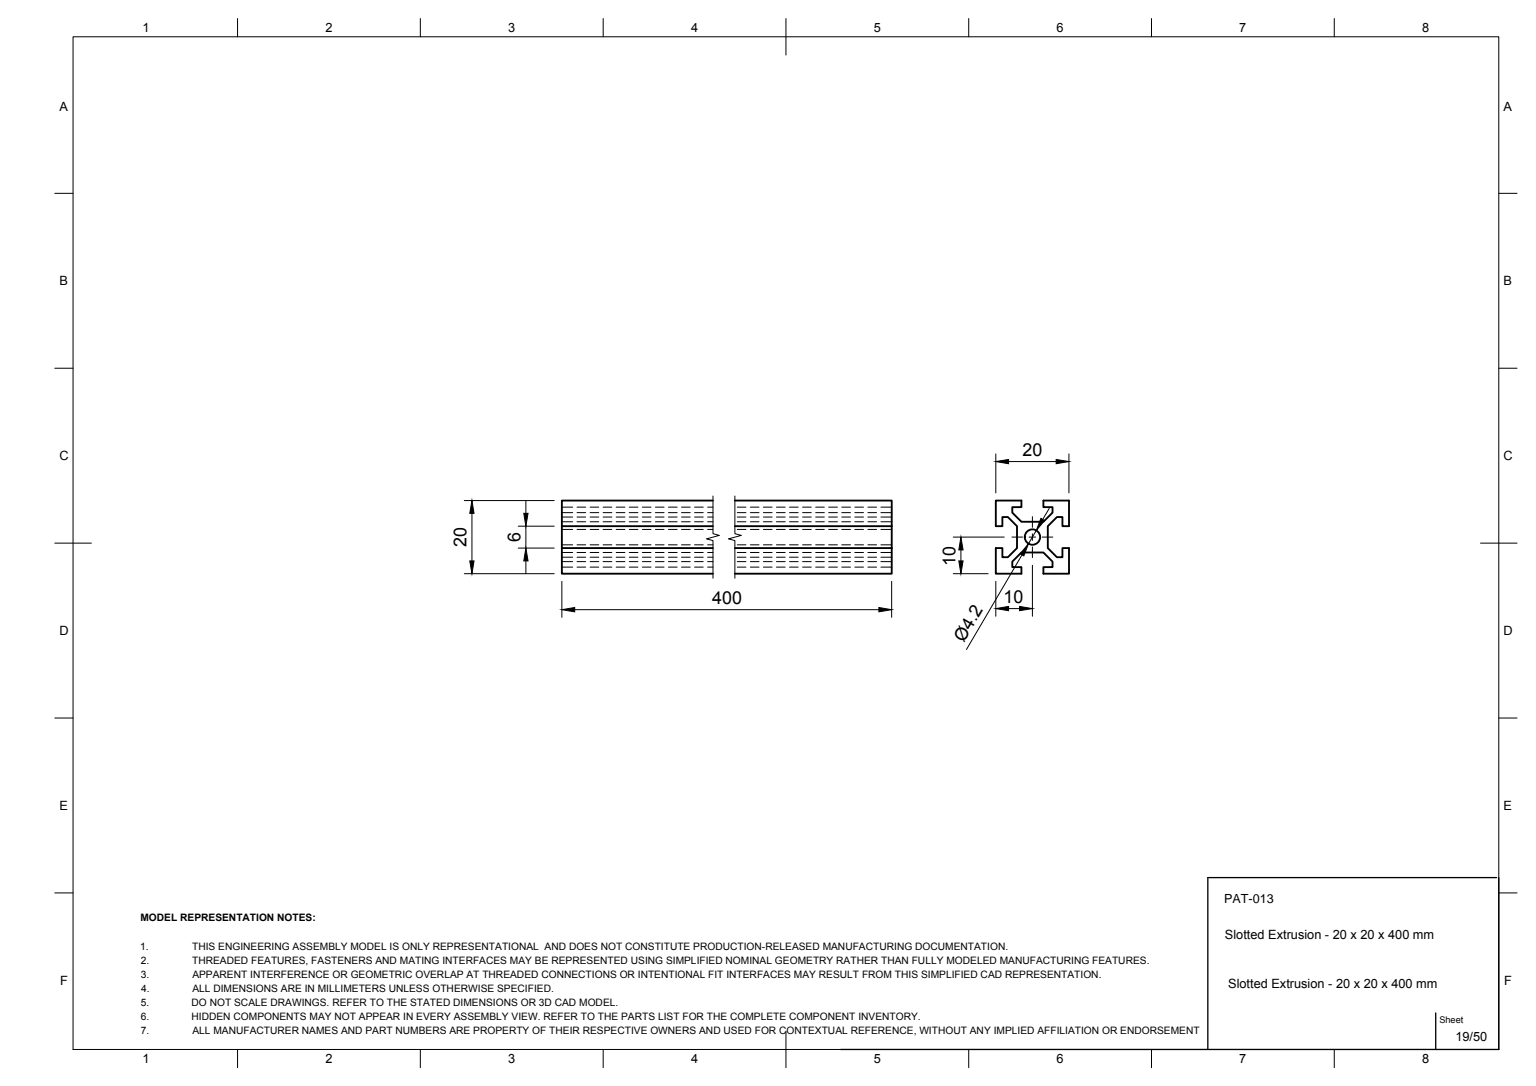
ISO-10303-21;
HEADER;
/* Generated by software containing ST-Developer
 * from STEP Tools, Inc. (www.steptools.com) 
 */

FILE_DESCRIPTION(
/* description */ ('Belt-driven linear axis on 2020 extrusion'),
/* implementation_level */ '2;1');

FILE_NAME(
/* name */ 'Slotted Extrusion - 20 x 20 x 400 mm.step',
/* time_stamp */ '2026-10-28T03:26:09-07:00',
/* author */ (''),
/* organization */ (''),
/* preprocessor_version */ 'ST-DEVELOPER v20.2',
/* originating_system */ 'Autodesk Translation Framework v15.17.0.0',
/* authorisation */ '');

FILE_SCHEMA (('AUTOMOTIVE_DESIGN { 1 0 10303 214 3 1 1 }'));
ENDSEC;

DATA;
#10=MECHANICAL_DESIGN_GEOMETRIC_PRESENTATION_REPRESENTATION('',(#639),#20096);
#537=SHAPE_REPRESENTATION_RELATIONSHIP('SRR','None',#20334,#583);
#583=ADVANCED_BREP_SHAPE_REPRESENTATION('',(#695),#20065);
#639=STYLED_ITEM('',(#20636),#695);
#695=MANIFOLD_SOLID_BREP('Body1',#10952);
#813=FACE_BOUND('',#2278,.T.);
#814=FACE_BOUND('',#2280,.T.);
#1022=PLANE('',#12051);
#1023=PLANE('',#12052);
#1024=PLANE('',#12053);
#1025=PLANE('',#12054);
#1026=PLANE('',#12055);
#1027=PLANE('',#12056);
#1028=PLANE('',#12057);
#1029=PLANE('',#12058);
#1030=PLANE('',#12059);
#1031=PLANE('',#12060);
#1032=PLANE('',#12061);
#1033=PLANE('',#12062);
#1034=PLANE('',#12063);
#1035=PLANE('',#12064);
#1036=PLANE('',#12065);
#1037=PLANE('',#12066);
#1038=PLANE('',#12067);
#1039=PLANE('',#12068);
#1040=PLANE('',#12069);
#1041=PLANE('',#12070);
#1042=PLANE('',#12071);
#1043=PLANE('',#12072);
#1044=PLANE('',#12073);
#1045=PLANE('',#12074);
#1046=PLANE('',#12075);
#1047=PLANE('',#12076);
#1048=PLANE('',#12077);
#1049=PLANE('',#12078);
#1050=PLANE('',#12079);
#1051=PLANE('',#12080);
#1052=PLANE('',#12081);
#1053=PLANE('',#12082);
#1054=PLANE('',#12083);
#1055=PLANE('',#12084);
#1056=PLANE('',#12085);
#1057=PLANE('',#12086);
#1058=PLANE('',#12090);
#1059=PLANE('',#12091);
#1060=PLANE('',#12092);
#1061=PLANE('',#12093);
#1062=PLANE('',#12094);
#1063=PLANE('',#12095);
#1064=PLANE('',#12096);
#1065=PLANE('',#12097);
#1066=PLANE('',#12098);
#1067=PLANE('',#12099);
#1515=FACE_OUTER_BOUND('',#2232,.T.);
#1516=FACE_OUTER_BOUND('',#2233,.T.);
#1517=FACE_OUTER_BOUND('',#2234,.T.);
#1518=FACE_OUTER_BOUND('',#2235,.T.);
#1519=FACE_OUTER_BOUND('',#2236,.T.);
#1520=FACE_OUTER_BOUND('',#2237,.T.);
#1521=FACE_OUTER_BOUND('',#2238,.T.);
#1522=FACE_OUTER_BOUND('',#2239,.T.);
#1523=FACE_OUTER_BOUND('',#2240,.T.);
#1524=FACE_OUTER_BOUND('',#2241,.T.);
#1525=FACE_OUTER_BOUND('',#2242,.T.);
#1526=FACE_OUTER_BOUND('',#2243,.T.);
#1527=FACE_OUTER_BOUND('',#2244,.T.);
#1528=FACE_OUTER_BOUND('',#2245,.T.);
#1529=FACE_OUTER_BOUND('',#2246,.T.);
#1530=FACE_OUTER_BOUND('',#2247,.T.);
#1531=FACE_OUTER_BOUND('',#2248,.T.);
#1532=FACE_OUTER_BOUND('',#2249,.T.);
#1533=FACE_OUTER_BOUND('',#2250,.T.);
#1534=FACE_OUTER_BOUND('',#2251,.T.);
#1535=FACE_OUTER_BOUND('',#2252,.T.);
#1536=FACE_OUTER_BOUND('',#2253,.T.);
#1537=FACE_OUTER_BOUND('',#2254,.T.);
#1538=FACE_OUTER_BOUND('',#2255,.T.);
#1539=FACE_OUTER_BOUND('',#2256,.T.);
#1540=FACE_OUTER_BOUND('',#2257,.T.);
#1541=FACE_OUTER_BOUND('',#2258,.T.);
#1542=FACE_OUTER_BOUND('',#2259,.T.);
#1543=FACE_OUTER_BOUND('',#2260,.T.);
#1544=FACE_OUTER_BOUND('',#2261,.T.);
#1545=FACE_OUTER_BOUND('',#2262,.T.);
#1546=FACE_OUTER_BOUND('',#2263,.T.);
#1547=FACE_OUTER_BOUND('',#2264,.T.);
#1548=FACE_OUTER_BOUND('',#2265,.T.);
#1549=FACE_OUTER_BOUND('',#2266,.T.);
#1550=FACE_OUTER_BOUND('',#2267,.T.);
#1551=FACE_OUTER_BOUND('',#2268,.T.);
#1552=FACE_OUTER_BOUND('',#2269,.T.);
#1553=FACE_OUTER_BOUND('',#2270,.T.);
#1554=FACE_OUTER_BOUND('',#2271,.T.);
#1555=FACE_OUTER_BOUND('',#2272,.T.);
#1556=FACE_OUTER_BOUND('',#2273,.T.);
#1557=FACE_OUTER_BOUND('',#2274,.T.);
#1558=FACE_OUTER_BOUND('',#2275,.T.);
#1559=FACE_OUTER_BOUND('',#2276,.T.);
#1560=FACE_OUTER_BOUND('',#2277,.T.);
#1561=FACE_OUTER_BOUND('',#2279,.T.);
#2232=EDGE_LOOP('',(#8437,#8438,#8439,#8440));
#2233=EDGE_LOOP('',(#8441,#8442,#8443,#8444));
#2234=EDGE_LOOP('',(#8445,#8446,#8447,#8448));
#2235=EDGE_LOOP('',(#8449,#8450,#8451,#8452));
#2236=EDGE_LOOP('',(#8453,#8454,#8455,#8456));
#2237=EDGE_LOOP('',(#8457,#8458,#8459,#8460));
#2238=EDGE_LOOP('',(#8461,#8462,#8463,#8464));
#2239=EDGE_LOOP('',(#8465,#8466,#8467,#8468));
#2240=EDGE_LOOP('',(#8469,#8470,#8471,#8472));
#2241=EDGE_LOOP('',(#8473,#8474,#8475,#8476));
#2242=EDGE_LOOP('',(#8477,#8478,#8479,#8480));
#2243=EDGE_LOOP('',(#8481,#8482,#8483,#8484));
#2244=EDGE_LOOP('',(#8485,#8486,#8487,#8488));
#2245=EDGE_LOOP('',(#8489,#8490,#8491,#8492));
#2246=EDGE_LOOP('',(#8493,#8494,#8495,#8496));
#2247=EDGE_LOOP('',(#8497,#8498,#8499,#8500));
#2248=EDGE_LOOP('',(#8501,#8502,#8503,#8504));
#2249=EDGE_LOOP('',(#8505,#8506,#8507,#8508));
#2250=EDGE_LOOP('',(#8509,#8510,#8511,#8512));
#2251=EDGE_LOOP('',(#8513,#8514,#8515,#8516));
#2252=EDGE_LOOP('',(#8517,#8518,#8519,#8520));
#2253=EDGE_LOOP('',(#8521,#8522,#8523,#8524));
#2254=EDGE_LOOP('',(#8525,#8526,#8527,#8528));
#2255=EDGE_LOOP('',(#8529,#8530,#8531,#8532));
#2256=EDGE_LOOP('',(#8533,#8534,#8535,#8536));
#2257=EDGE_LOOP('',(#8537,#8538,#8539,#8540));
#2258=EDGE_LOOP('',(#8541,#8542,#8543,#8544));
#2259=EDGE_LOOP('',(#8545,#8546,#8547,#8548));
#2260=EDGE_LOOP('',(#8549,#8550,#8551,#8552));
#2261=EDGE_LOOP('',(#8553,#8554,#8555,#8556));
#2262=EDGE_LOOP('',(#8557,#8558,#8559,#8560));
#2263=EDGE_LOOP('',(#8561,#8562,#8563,#8564));
#2264=EDGE_LOOP('',(#8565,#8566,#8567,#8568));
#2265=EDGE_LOOP('',(#8569,#8570,#8571,#8572));
#2266=EDGE_LOOP('',(#8573,#8574,#8575,#8576));
#2267=EDGE_LOOP('',(#8577,#8578,#8579,#8580));
#2268=EDGE_LOOP('',(#8581,#8582,#8583,#8584));
#2269=EDGE_LOOP('',(#8585,#8586,#8587,#8588));
#2270=EDGE_LOOP('',(#8589,#8590,#8591,#8592));
#2271=EDGE_LOOP('',(#8593,#8594,#8595,#8596));
#2272=EDGE_LOOP('',(#8597,#8598,#8599,#8600));
#2273=EDGE_LOOP('',(#8601,#8602,#8603,#8604));
#2274=EDGE_LOOP('',(#8605,#8606,#8607,#8608));
#2275=EDGE_LOOP('',(#8609,#8610,#8611,#8612));
#2276=EDGE_LOOP('',(#8613,#8614,#8615,#8616));
#2277=EDGE_LOOP('',(#8617,#8618,#8619,#8620,#8621,#8622,#8623,#8624,#8625,
#8626,#8627,#8628,#8629,#8630,#8631,#8632,#8633,#8634,#8635,#8636,#8637,
#8638,#8639,#8640,#8641,#8642,#8643,#8644,#8645,#8646,#8647,#8648,#8649,
#8650,#8651,#8652,#8653,#8654,#8655,#8656,#8657,#8658,#8659,#8660));
#2278=EDGE_LOOP('',(#8661));
#2279=EDGE_LOOP('',(#8662,#8663,#8664,#8665,#8666,#8667,#8668,#8669,#8670,
#8671,#8672,#8673,#8674,#8675,#8676,#8677,#8678,#8679,#8680,#8681,#8682,
#8683,#8684,#8685,#8686,#8687,#8688,#8689,#8690,#8691,#8692,#8693,#8694,
#8695,#8696,#8697,#8698,#8699,#8700,#8701,#8702,#8703,#8704,#8705));
#2280=EDGE_LOOP('',(#8706));
#2971=LINE('',#17862,#3828);
#2972=LINE('',#17864,#3829);
#2973=LINE('',#17866,#3830);
#2974=LINE('',#17867,#3831);
#2975=LINE('',#17870,#3832);
#2976=LINE('',#17872,#3833);
#2977=LINE('',#17873,#3834);
#2978=LINE('',#17876,#3835);
#2979=LINE('',#17878,#3836);
#2980=LINE('',#17879,#3837);
#2981=LINE('',#17882,#3838);
#2982=LINE('',#17884,#3839);
#2983=LINE('',#17885,#3840);
#2984=LINE('',#17888,#3841);
#2985=LINE('',#17890,#3842);
#2986=LINE('',#17891,#3843);
#2987=LINE('',#17894,#3844);
#2988=LINE('',#17896,#3845);
#2989=LINE('',#17897,#3846);
#2990=LINE('',#17900,#3847);
#2991=LINE('',#17902,#3848);
#2992=LINE('',#17903,#3849);
#2993=LINE('',#17906,#3850);
#2994=LINE('',#17908,#3851);
#2995=LINE('',#17909,#3852);
#2996=LINE('',#17912,#3853);
#2997=LINE('',#17914,#3854);
#2998=LINE('',#17915,#3855);
#2999=LINE('',#17919,#3856);
#3000=LINE('',#17921,#3857);
#3001=LINE('',#17923,#3858);
#3002=LINE('',#17924,#3859);
#3003=LINE('',#17927,#3860);
#3004=LINE('',#17929,#3861);
#3005=LINE('',#17930,#3862);
#3006=LINE('',#17933,#3863);
#3007=LINE('',#17935,#3864);
#3008=LINE('',#17936,#3865);
#3009=LINE('',#17939,#3866);
#3010=LINE('',#17941,#3867);
#3011=LINE('',#17942,#3868);
#3012=LINE('',#17945,#3869);
#3013=LINE('',#17947,#3870);
#3014=LINE('',#17948,#3871);
#3015=LINE('',#17951,#3872);
#3016=LINE('',#17953,#3873);
#3017=LINE('',#17954,#3874);
#3018=LINE('',#17957,#3875);
#3019=LINE('',#17959,#3876);
#3020=LINE('',#17960,#3877);
#3021=LINE('',#17963,#3878);
#3022=LINE('',#17965,#3879);
#3023=LINE('',#17966,#3880);
#3024=LINE('',#17969,#3881);
#3025=LINE('',#17971,#3882);
#3026=LINE('',#17972,#3883);
#3027=LINE('',#17976,#3884);
#3028=LINE('',#17978,#3885);
#3029=LINE('',#17980,#3886);
#3030=LINE('',#17981,#3887);
#3031=LINE('',#17984,#3888);
#3032=LINE('',#17986,#3889);
#3033=LINE('',#17987,#3890);
#3034=LINE('',#17990,#3891);
#3035=LINE('',#17992,#3892);
#3036=LINE('',#17993,#3893);
#3037=LINE('',#17996,#3894);
#3038=LINE('',#17998,#3895);
#3039=LINE('',#17999,#3896);
#3040=LINE('',#18002,#3897);
#3041=LINE('',#18004,#3898);
#3042=LINE('',#18005,#3899);
#3043=LINE('',#18008,#3900);
#3044=LINE('',#18010,#3901);
#3045=LINE('',#18011,#3902);
#3046=LINE('',#18014,#3903);
#3047=LINE('',#18016,#3904);
#3048=LINE('',#18017,#3905);
#3049=LINE('',#18020,#3906);
#3050=LINE('',#18022,#3907);
#3051=LINE('',#18023,#3908);
#3052=LINE('',#18026,#3909);
#3053=LINE('',#18028,#3910);
#3054=LINE('',#18029,#3911);
#3055=LINE('',#18033,#3912);
#3056=LINE('',#18035,#3913);
#3057=LINE('',#18037,#3914);
#3058=LINE('',#18038,#3915);
#3059=LINE('',#18041,#3916);
#3060=LINE('',#18043,#3917);
#3061=LINE('',#18044,#3918);
#3062=LINE('',#18047,#3919);
#3063=LINE('',#18049,#3920);
#3064=LINE('',#18050,#3921);
#3065=LINE('',#18053,#3922);
#3066=LINE('',#18055,#3923);
#3067=LINE('',#18056,#3924);
#3068=LINE('',#18059,#3925);
#3069=LINE('',#18061,#3926);
#3070=LINE('',#18062,#3927);
#3071=LINE('',#18065,#3928);
#3072=LINE('',#18067,#3929);
#3073=LINE('',#18068,#3930);
#3074=LINE('',#18071,#3931);
#3075=LINE('',#18073,#3932);
#3076=LINE('',#18074,#3933);
#3077=LINE('',#18077,#3934);
#3078=LINE('',#18079,#3935);
#3079=LINE('',#18080,#3936);
#3080=LINE('',#18083,#3937);
#3081=LINE('',#18085,#3938);
#3082=LINE('',#18086,#3939);
#3083=LINE('',#18091,#3940);
#3084=LINE('',#18095,#3941);
#3085=LINE('',#18097,#3942);
#3086=LINE('',#18098,#3943);
#3087=LINE('',#18101,#3944);
#3088=LINE('',#18103,#3945);
#3089=LINE('',#18104,#3946);
#3090=LINE('',#18106,#3947);
#3091=LINE('',#18107,#3948);
#3092=LINE('',#18110,#3949);
#3093=LINE('',#18112,#3950);
#3094=LINE('',#18113,#3951);
#3095=LINE('',#18115,#3952);
#3096=LINE('',#18116,#3953);
#3097=LINE('',#18119,#3954);
#3098=LINE('',#18121,#3955);
#3099=LINE('',#18122,#3956);
#3100=LINE('',#18124,#3957);
#3101=LINE('',#18125,#3958);
#3102=LINE('',#18127,#3959);
#3103=LINE('',#18128,#3960);
#3828=VECTOR('',#14215,1.);
#3829=VECTOR('',#14216,1.);
#3830=VECTOR('',#14217,1.);
#3831=VECTOR('',#14218,1.);
#3832=VECTOR('',#14221,1.);
#3833=VECTOR('',#14222,1.);
#3834=VECTOR('',#14223,1.);
#3835=VECTOR('',#14226,1.);
#3836=VECTOR('',#14227,1.);
#3837=VECTOR('',#14228,1.);
#3838=VECTOR('',#14231,1.);
#3839=VECTOR('',#14232,1.);
#3840=VECTOR('',#14233,1.);
#3841=VECTOR('',#14236,1.);
#3842=VECTOR('',#14237,1.);
#3843=VECTOR('',#14238,1.);
#3844=VECTOR('',#14241,1.);
#3845=VECTOR('',#14242,1.);
#3846=VECTOR('',#14243,1.);
#3847=VECTOR('',#14246,1.);
#3848=VECTOR('',#14247,1.);
#3849=VECTOR('',#14248,1.);
#3850=VECTOR('',#14251,1.);
#3851=VECTOR('',#14252,1.);
#3852=VECTOR('',#14253,1.);
#3853=VECTOR('',#14256,1.);
#3854=VECTOR('',#14257,1.);
#3855=VECTOR('',#14258,1.);
#3856=VECTOR('',#14261,1.);
#3857=VECTOR('',#14262,1.);
#3858=VECTOR('',#14263,1.);
#3859=VECTOR('',#14264,1.);
#3860=VECTOR('',#14267,1.);
#3861=VECTOR('',#14268,1.);
#3862=VECTOR('',#14269,1.);
#3863=VECTOR('',#14272,1.);
#3864=VECTOR('',#14273,1.);
#3865=VECTOR('',#14274,1.);
#3866=VECTOR('',#14277,1.);
#3867=VECTOR('',#14278,1.);
#3868=VECTOR('',#14279,1.);
#3869=VECTOR('',#14282,1.);
#3870=VECTOR('',#14283,1.);
#3871=VECTOR('',#14284,1.);
#3872=VECTOR('',#14287,1.);
#3873=VECTOR('',#14288,1.);
#3874=VECTOR('',#14289,1.);
#3875=VECTOR('',#14292,1.);
#3876=VECTOR('',#14293,1.);
#3877=VECTOR('',#14294,1.);
#3878=VECTOR('',#14297,1.);
#3879=VECTOR('',#14298,1.);
#3880=VECTOR('',#14299,1.);
#3881=VECTOR('',#14302,1.);
#3882=VECTOR('',#14303,1.);
#3883=VECTOR('',#14304,1.);
#3884=VECTOR('',#14307,1.);
#3885=VECTOR('',#14308,1.);
#3886=VECTOR('',#14309,1.);
#3887=VECTOR('',#14310,1.);
#3888=VECTOR('',#14313,1.);
#3889=VECTOR('',#14314,1.);
#3890=VECTOR('',#14315,1.);
#3891=VECTOR('',#14318,1.);
#3892=VECTOR('',#14319,1.);
#3893=VECTOR('',#14320,1.);
#3894=VECTOR('',#14323,1.);
#3895=VECTOR('',#14324,1.);
#3896=VECTOR('',#14325,1.);
#3897=VECTOR('',#14328,1.);
#3898=VECTOR('',#14329,1.);
#3899=VECTOR('',#14330,1.);
#3900=VECTOR('',#14333,1.);
#3901=VECTOR('',#14334,1.);
#3902=VECTOR('',#14335,1.);
#3903=VECTOR('',#14338,1.);
#3904=VECTOR('',#14339,1.);
#3905=VECTOR('',#14340,1.);
#3906=VECTOR('',#14343,1.);
#3907=VECTOR('',#14344,1.);
#3908=VECTOR('',#14345,1.);
#3909=VECTOR('',#14348,1.);
#3910=VECTOR('',#14349,1.);
#3911=VECTOR('',#14350,1.);
#3912=VECTOR('',#14353,1.);
#3913=VECTOR('',#14354,1.);
#3914=VECTOR('',#14355,1.);
#3915=VECTOR('',#14356,1.);
#3916=VECTOR('',#14359,1.);
#3917=VECTOR('',#14360,1.);
#3918=VECTOR('',#14361,1.);
#3919=VECTOR('',#14364,1.);
#3920=VECTOR('',#14365,1.);
#3921=VECTOR('',#14366,1.);
#3922=VECTOR('',#14369,1.);
#3923=VECTOR('',#14370,1.);
#3924=VECTOR('',#14371,1.);
#3925=VECTOR('',#14374,1.);
#3926=VECTOR('',#14375,1.);
#3927=VECTOR('',#14376,1.);
#3928=VECTOR('',#14379,1.);
#3929=VECTOR('',#14380,1.);
#3930=VECTOR('',#14381,1.);
#3931=VECTOR('',#14384,1.);
#3932=VECTOR('',#14385,1.);
#3933=VECTOR('',#14386,1.);
#3934=VECTOR('',#14389,1.);
#3935=VECTOR('',#14390,1.);
#3936=VECTOR('',#14391,1.);
#3937=VECTOR('',#14394,1.);
#3938=VECTOR('',#14395,1.);
#3939=VECTOR('',#14396,1.);
#3940=VECTOR('',#14401,0.21);
#3941=VECTOR('',#14406,1.);
#3942=VECTOR('',#14407,1.);
#3943=VECTOR('',#14408,1.);
#3944=VECTOR('',#14411,1.);
#3945=VECTOR('',#14412,1.);
#3946=VECTOR('',#14413,1.);
#3947=VECTOR('',#14416,1.);
#3948=VECTOR('',#14417,1.);
#3949=VECTOR('',#14420,1.);
#3950=VECTOR('',#14421,1.);
#3951=VECTOR('',#14422,1.);
#3952=VECTOR('',#14425,1.);
#3953=VECTOR('',#14426,1.);
#3954=VECTOR('',#14429,1.);
#3955=VECTOR('',#14430,1.);
#3956=VECTOR('',#14431,1.);
#3957=VECTOR('',#14434,1.);
#3958=VECTOR('',#14435,1.);
#3959=VECTOR('',#14438,1.);
#3960=VECTOR('',#14439,1.);
#4647=CIRCLE('',#12088,0.21);
#4648=CIRCLE('',#12089,0.21);
#5296=VERTEX_POINT('',#17860);
#5297=VERTEX_POINT('',#17861);
#5298=VERTEX_POINT('',#17863);
#5299=VERTEX_POINT('',#17865);
#5300=VERTEX_POINT('',#17869);
#5301=VERTEX_POINT('',#17871);
#5302=VERTEX_POINT('',#17875);
#5303=VERTEX_POINT('',#17877);
#5304=VERTEX_POINT('',#17881);
#5305=VERTEX_POINT('',#17883);
#5306=VERTEX_POINT('',#17887);
#5307=VERTEX_POINT('',#17889);
#5308=VERTEX_POINT('',#17893);
#5309=VERTEX_POINT('',#17895);
#5310=VERTEX_POINT('',#17899);
#5311=VERTEX_POINT('',#17901);
#5312=VERTEX_POINT('',#17905);
#5313=VERTEX_POINT('',#17907);
#5314=VERTEX_POINT('',#17911);
#5315=VERTEX_POINT('',#17913);
#5316=VERTEX_POINT('',#17917);
#5317=VERTEX_POINT('',#17918);
#5318=VERTEX_POINT('',#17920);
#5319=VERTEX_POINT('',#17922);
#5320=VERTEX_POINT('',#17926);
#5321=VERTEX_POINT('',#17928);
#5322=VERTEX_POINT('',#17932);
#5323=VERTEX_POINT('',#17934);
#5324=VERTEX_POINT('',#17938);
#5325=VERTEX_POINT('',#17940);
#5326=VERTEX_POINT('',#17944);
#5327=VERTEX_POINT('',#17946);
#5328=VERTEX_POINT('',#17950);
#5329=VERTEX_POINT('',#17952);
#5330=VERTEX_POINT('',#17956);
#5331=VERTEX_POINT('',#17958);
#5332=VERTEX_POINT('',#17962);
#5333=VERTEX_POINT('',#17964);
#5334=VERTEX_POINT('',#17968);
#5335=VERTEX_POINT('',#17970);
#5336=VERTEX_POINT('',#17974);
#5337=VERTEX_POINT('',#17975);
#5338=VERTEX_POINT('',#17977);
#5339=VERTEX_POINT('',#17979);
#5340=VERTEX_POINT('',#17983);
#5341=VERTEX_POINT('',#17985);
#5342=VERTEX_POINT('',#17989);
#5343=VERTEX_POINT('',#17991);
#5344=VERTEX_POINT('',#17995);
#5345=VERTEX_POINT('',#17997);
#5346=VERTEX_POINT('',#18001);
#5347=VERTEX_POINT('',#18003);
#5348=VERTEX_POINT('',#18007);
#5349=VERTEX_POINT('',#18009);
#5350=VERTEX_POINT('',#18013);
#5351=VERTEX_POINT('',#18015);
#5352=VERTEX_POINT('',#18019);
#5353=VERTEX_POINT('',#18021);
#5354=VERTEX_POINT('',#18025);
#5355=VERTEX_POINT('',#18027);
#5356=VERTEX_POINT('',#18031);
#5357=VERTEX_POINT('',#18032);
#5358=VERTEX_POINT('',#18034);
#5359=VERTEX_POINT('',#18036);
#5360=VERTEX_POINT('',#18040);
#5361=VERTEX_POINT('',#18042);
#5362=VERTEX_POINT('',#18046);
#5363=VERTEX_POINT('',#18048);
#5364=VERTEX_POINT('',#18052);
#5365=VERTEX_POINT('',#18054);
#5366=VERTEX_POINT('',#18058);
#5367=VERTEX_POINT('',#18060);
#5368=VERTEX_POINT('',#18064);
#5369=VERTEX_POINT('',#18066);
#5370=VERTEX_POINT('',#18070);
#5371=VERTEX_POINT('',#18072);
#5372=VERTEX_POINT('',#18076);
#5373=VERTEX_POINT('',#18078);
#5374=VERTEX_POINT('',#18082);
#5375=VERTEX_POINT('',#18084);
#5376=VERTEX_POINT('',#18088);
#5377=VERTEX_POINT('',#18090);
#5378=VERTEX_POINT('',#18094);
#5379=VERTEX_POINT('',#18096);
#5380=VERTEX_POINT('',#18100);
#5381=VERTEX_POINT('',#18102);
#5382=VERTEX_POINT('',#18109);
#5383=VERTEX_POINT('',#18111);
#5384=VERTEX_POINT('',#18118);
#5385=VERTEX_POINT('',#18120);
#6433=EDGE_CURVE('',#5296,#5297,#2971,.T.);
#6434=EDGE_CURVE('',#5296,#5298,#2972,.T.);
#6435=EDGE_CURVE('',#5299,#5298,#2973,.T.);
#6436=EDGE_CURVE('',#5297,#5299,#2974,.T.);
#6437=EDGE_CURVE('',#5300,#5296,#2975,.T.);
#6438=EDGE_CURVE('',#5300,#5301,#2976,.T.);
#6439=EDGE_CURVE('',#5298,#5301,#2977,.T.);
#6440=EDGE_CURVE('',#5302,#5300,#2978,.T.);
#6441=EDGE_CURVE('',#5302,#5303,#2979,.T.);
#6442=EDGE_CURVE('',#5301,#5303,#2980,.T.);
#6443=EDGE_CURVE('',#5304,#5302,#2981,.T.);
#6444=EDGE_CURVE('',#5304,#5305,#2982,.T.);
#6445=EDGE_CURVE('',#5303,#5305,#2983,.T.);
#6446=EDGE_CURVE('',#5306,#5304,#2984,.T.);
#6447=EDGE_CURVE('',#5306,#5307,#2985,.T.);
#6448=EDGE_CURVE('',#5305,#5307,#2986,.T.);
#6449=EDGE_CURVE('',#5308,#5306,#2987,.T.);
#6450=EDGE_CURVE('',#5308,#5309,#2988,.T.);
#6451=EDGE_CURVE('',#5307,#5309,#2989,.T.);
#6452=EDGE_CURVE('',#5310,#5308,#2990,.T.);
#6453=EDGE_CURVE('',#5310,#5311,#2991,.T.);
#6454=EDGE_CURVE('',#5309,#5311,#2992,.T.);
#6455=EDGE_CURVE('',#5312,#5310,#2993,.T.);
#6456=EDGE_CURVE('',#5312,#5313,#2994,.T.);
#6457=EDGE_CURVE('',#5311,#5313,#2995,.T.);
#6458=EDGE_CURVE('',#5314,#5312,#2996,.T.);
#6459=EDGE_CURVE('',#5315,#5314,#2997,.T.);
#6460=EDGE_CURVE('',#5313,#5315,#2998,.T.);
#6461=EDGE_CURVE('',#5316,#5317,#2999,.T.);
#6462=EDGE_CURVE('',#5316,#5318,#3000,.T.);
#6463=EDGE_CURVE('',#5319,#5318,#3001,.T.);
#6464=EDGE_CURVE('',#5317,#5319,#3002,.T.);
#6465=EDGE_CURVE('',#5320,#5316,#3003,.T.);
#6466=EDGE_CURVE('',#5320,#5321,#3004,.T.);
#6467=EDGE_CURVE('',#5318,#5321,#3005,.T.);
#6468=EDGE_CURVE('',#5322,#5320,#3006,.T.);
#6469=EDGE_CURVE('',#5322,#5323,#3007,.T.);
#6470=EDGE_CURVE('',#5321,#5323,#3008,.T.);
#6471=EDGE_CURVE('',#5324,#5322,#3009,.T.);
#6472=EDGE_CURVE('',#5324,#5325,#3010,.T.);
#6473=EDGE_CURVE('',#5323,#5325,#3011,.T.);
#6474=EDGE_CURVE('',#5326,#5324,#3012,.T.);
#6475=EDGE_CURVE('',#5326,#5327,#3013,.T.);
#6476=EDGE_CURVE('',#5325,#5327,#3014,.T.);
#6477=EDGE_CURVE('',#5328,#5326,#3015,.T.);
#6478=EDGE_CURVE('',#5328,#5329,#3016,.T.);
#6479=EDGE_CURVE('',#5327,#5329,#3017,.T.);
#6480=EDGE_CURVE('',#5330,#5328,#3018,.T.);
#6481=EDGE_CURVE('',#5330,#5331,#3019,.T.);
#6482=EDGE_CURVE('',#5329,#5331,#3020,.T.);
#6483=EDGE_CURVE('',#5332,#5330,#3021,.T.);
#6484=EDGE_CURVE('',#5332,#5333,#3022,.T.);
#6485=EDGE_CURVE('',#5331,#5333,#3023,.T.);
#6486=EDGE_CURVE('',#5334,#5332,#3024,.T.);
#6487=EDGE_CURVE('',#5335,#5334,#3025,.T.);
#6488=EDGE_CURVE('',#5333,#5335,#3026,.T.);
#6489=EDGE_CURVE('',#5336,#5337,#3027,.T.);
#6490=EDGE_CURVE('',#5336,#5338,#3028,.T.);
#6491=EDGE_CURVE('',#5339,#5338,#3029,.T.);
#6492=EDGE_CURVE('',#5337,#5339,#3030,.T.);
#6493=EDGE_CURVE('',#5340,#5336,#3031,.T.);
#6494=EDGE_CURVE('',#5340,#5341,#3032,.T.);
#6495=EDGE_CURVE('',#5338,#5341,#3033,.T.);
#6496=EDGE_CURVE('',#5342,#5340,#3034,.T.);
#6497=EDGE_CURVE('',#5342,#5343,#3035,.T.);
#6498=EDGE_CURVE('',#5341,#5343,#3036,.T.);
#6499=EDGE_CURVE('',#5344,#5342,#3037,.T.);
#6500=EDGE_CURVE('',#5344,#5345,#3038,.T.);
#6501=EDGE_CURVE('',#5343,#5345,#3039,.T.);
#6502=EDGE_CURVE('',#5346,#5344,#3040,.T.);
#6503=EDGE_CURVE('',#5346,#5347,#3041,.T.);
#6504=EDGE_CURVE('',#5345,#5347,#3042,.T.);
#6505=EDGE_CURVE('',#5348,#5346,#3043,.T.);
#6506=EDGE_CURVE('',#5348,#5349,#3044,.T.);
#6507=EDGE_CURVE('',#5347,#5349,#3045,.T.);
#6508=EDGE_CURVE('',#5350,#5348,#3046,.T.);
#6509=EDGE_CURVE('',#5350,#5351,#3047,.T.);
#6510=EDGE_CURVE('',#5349,#5351,#3048,.T.);
#6511=EDGE_CURVE('',#5352,#5350,#3049,.T.);
#6512=EDGE_CURVE('',#5352,#5353,#3050,.T.);
#6513=EDGE_CURVE('',#5351,#5353,#3051,.T.);
#6514=EDGE_CURVE('',#5354,#5352,#3052,.T.);
#6515=EDGE_CURVE('',#5355,#5354,#3053,.T.);
#6516=EDGE_CURVE('',#5353,#5355,#3054,.T.);
#6517=EDGE_CURVE('',#5356,#5357,#3055,.T.);
#6518=EDGE_CURVE('',#5356,#5358,#3056,.T.);
#6519=EDGE_CURVE('',#5359,#5358,#3057,.T.);
#6520=EDGE_CURVE('',#5357,#5359,#3058,.T.);
#6521=EDGE_CURVE('',#5360,#5356,#3059,.T.);
#6522=EDGE_CURVE('',#5360,#5361,#3060,.T.);
#6523=EDGE_CURVE('',#5358,#5361,#3061,.T.);
#6524=EDGE_CURVE('',#5362,#5360,#3062,.T.);
#6525=EDGE_CURVE('',#5362,#5363,#3063,.T.);
#6526=EDGE_CURVE('',#5361,#5363,#3064,.T.);
#6527=EDGE_CURVE('',#5364,#5362,#3065,.T.);
#6528=EDGE_CURVE('',#5364,#5365,#3066,.T.);
#6529=EDGE_CURVE('',#5363,#5365,#3067,.T.);
#6530=EDGE_CURVE('',#5366,#5364,#3068,.T.);
#6531=EDGE_CURVE('',#5366,#5367,#3069,.T.);
#6532=EDGE_CURVE('',#5365,#5367,#3070,.T.);
#6533=EDGE_CURVE('',#5368,#5366,#3071,.T.);
#6534=EDGE_CURVE('',#5368,#5369,#3072,.T.);
#6535=EDGE_CURVE('',#5367,#5369,#3073,.T.);
#6536=EDGE_CURVE('',#5370,#5368,#3074,.T.);
#6537=EDGE_CURVE('',#5370,#5371,#3075,.T.);
#6538=EDGE_CURVE('',#5369,#5371,#3076,.T.);
#6539=EDGE_CURVE('',#5372,#5370,#3077,.T.);
#6540=EDGE_CURVE('',#5372,#5373,#3078,.T.);
#6541=EDGE_CURVE('',#5371,#5373,#3079,.T.);
#6542=EDGE_CURVE('',#5374,#5372,#3080,.T.);
#6543=EDGE_CURVE('',#5375,#5374,#3081,.T.);
#6544=EDGE_CURVE('',#5373,#5375,#3082,.T.);
#6545=EDGE_CURVE('',#5376,#5376,#4647,.T.);
#6546=EDGE_CURVE('',#5376,#5377,#3083,.T.);
#6547=EDGE_CURVE('',#5377,#5377,#4648,.T.);
#6548=EDGE_CURVE('',#5314,#5378,#3084,.T.);
#6549=EDGE_CURVE('',#5378,#5379,#3085,.T.);
#6550=EDGE_CURVE('',#5315,#5379,#3086,.T.);
#6551=EDGE_CURVE('',#5380,#5299,#3087,.T.);
#6552=EDGE_CURVE('',#5381,#5380,#3088,.T.);
#6553=EDGE_CURVE('',#5381,#5297,#3089,.T.);
#6554=EDGE_CURVE('',#5334,#5381,#3090,.T.);
#6555=EDGE_CURVE('',#5335,#5380,#3091,.T.);
#6556=EDGE_CURVE('',#5382,#5319,#3092,.T.);
#6557=EDGE_CURVE('',#5383,#5382,#3093,.T.);
#6558=EDGE_CURVE('',#5383,#5317,#3094,.T.);
#6559=EDGE_CURVE('',#5354,#5383,#3095,.T.);
#6560=EDGE_CURVE('',#5355,#5382,#3096,.T.);
#6561=EDGE_CURVE('',#5384,#5339,#3097,.T.);
#6562=EDGE_CURVE('',#5385,#5384,#3098,.T.);
#6563=EDGE_CURVE('',#5385,#5337,#3099,.T.);
#6564=EDGE_CURVE('',#5374,#5385,#3100,.T.);
#6565=EDGE_CURVE('',#5375,#5384,#3101,.T.);
#6566=EDGE_CURVE('',#5379,#5359,#3102,.T.);
#6567=EDGE_CURVE('',#5378,#5357,#3103,.T.);
#8437=ORIENTED_EDGE('',*,*,#6433,.F.);
#8438=ORIENTED_EDGE('',*,*,#6434,.T.);
#8439=ORIENTED_EDGE('',*,*,#6435,.F.);
#8440=ORIENTED_EDGE('',*,*,#6436,.F.);
#8441=ORIENTED_EDGE('',*,*,#6437,.F.);
#8442=ORIENTED_EDGE('',*,*,#6438,.T.);
#8443=ORIENTED_EDGE('',*,*,#6439,.F.);
#8444=ORIENTED_EDGE('',*,*,#6434,.F.);
#8445=ORIENTED_EDGE('',*,*,#6440,.F.);
#8446=ORIENTED_EDGE('',*,*,#6441,.T.);
#8447=ORIENTED_EDGE('',*,*,#6442,.F.);
#8448=ORIENTED_EDGE('',*,*,#6438,.F.);
#8449=ORIENTED_EDGE('',*,*,#6443,.F.);
#8450=ORIENTED_EDGE('',*,*,#6444,.T.);
#8451=ORIENTED_EDGE('',*,*,#6445,.F.);
#8452=ORIENTED_EDGE('',*,*,#6441,.F.);
#8453=ORIENTED_EDGE('',*,*,#6446,.F.);
#8454=ORIENTED_EDGE('',*,*,#6447,.T.);
#8455=ORIENTED_EDGE('',*,*,#6448,.F.);
#8456=ORIENTED_EDGE('',*,*,#6444,.F.);
#8457=ORIENTED_EDGE('',*,*,#6449,.F.);
#8458=ORIENTED_EDGE('',*,*,#6450,.T.);
#8459=ORIENTED_EDGE('',*,*,#6451,.F.);
#8460=ORIENTED_EDGE('',*,*,#6447,.F.);
#8461=ORIENTED_EDGE('',*,*,#6452,.F.);
#8462=ORIENTED_EDGE('',*,*,#6453,.T.);
#8463=ORIENTED_EDGE('',*,*,#6454,.F.);
#8464=ORIENTED_EDGE('',*,*,#6450,.F.);
#8465=ORIENTED_EDGE('',*,*,#6455,.F.);
#8466=ORIENTED_EDGE('',*,*,#6456,.T.);
#8467=ORIENTED_EDGE('',*,*,#6457,.F.);
#8468=ORIENTED_EDGE('',*,*,#6453,.F.);
#8469=ORIENTED_EDGE('',*,*,#6458,.F.);
#8470=ORIENTED_EDGE('',*,*,#6459,.F.);
#8471=ORIENTED_EDGE('',*,*,#6460,.F.);
#8472=ORIENTED_EDGE('',*,*,#6456,.F.);
#8473=ORIENTED_EDGE('',*,*,#6461,.F.);
#8474=ORIENTED_EDGE('',*,*,#6462,.T.);
#8475=ORIENTED_EDGE('',*,*,#6463,.F.);
#8476=ORIENTED_EDGE('',*,*,#6464,.F.);
#8477=ORIENTED_EDGE('',*,*,#6465,.F.);
#8478=ORIENTED_EDGE('',*,*,#6466,.T.);
#8479=ORIENTED_EDGE('',*,*,#6467,.F.);
#8480=ORIENTED_EDGE('',*,*,#6462,.F.);
#8481=ORIENTED_EDGE('',*,*,#6468,.F.);
#8482=ORIENTED_EDGE('',*,*,#6469,.T.);
#8483=ORIENTED_EDGE('',*,*,#6470,.F.);
#8484=ORIENTED_EDGE('',*,*,#6466,.F.);
#8485=ORIENTED_EDGE('',*,*,#6471,.F.);
#8486=ORIENTED_EDGE('',*,*,#6472,.T.);
#8487=ORIENTED_EDGE('',*,*,#6473,.F.);
#8488=ORIENTED_EDGE('',*,*,#6469,.F.);
#8489=ORIENTED_EDGE('',*,*,#6474,.F.);
#8490=ORIENTED_EDGE('',*,*,#6475,.T.);
#8491=ORIENTED_EDGE('',*,*,#6476,.F.);
#8492=ORIENTED_EDGE('',*,*,#6472,.F.);
#8493=ORIENTED_EDGE('',*,*,#6477,.F.);
#8494=ORIENTED_EDGE('',*,*,#6478,.T.);
#8495=ORIENTED_EDGE('',*,*,#6479,.F.);
#8496=ORIENTED_EDGE('',*,*,#6475,.F.);
#8497=ORIENTED_EDGE('',*,*,#6480,.F.);
#8498=ORIENTED_EDGE('',*,*,#6481,.T.);
#8499=ORIENTED_EDGE('',*,*,#6482,.F.);
#8500=ORIENTED_EDGE('',*,*,#6478,.F.);
#8501=ORIENTED_EDGE('',*,*,#6483,.F.);
#8502=ORIENTED_EDGE('',*,*,#6484,.T.);
#8503=ORIENTED_EDGE('',*,*,#6485,.F.);
#8504=ORIENTED_EDGE('',*,*,#6481,.F.);
#8505=ORIENTED_EDGE('',*,*,#6486,.F.);
#8506=ORIENTED_EDGE('',*,*,#6487,.F.);
#8507=ORIENTED_EDGE('',*,*,#6488,.F.);
#8508=ORIENTED_EDGE('',*,*,#6484,.F.);
#8509=ORIENTED_EDGE('',*,*,#6489,.F.);
#8510=ORIENTED_EDGE('',*,*,#6490,.T.);
#8511=ORIENTED_EDGE('',*,*,#6491,.F.);
#8512=ORIENTED_EDGE('',*,*,#6492,.F.);
#8513=ORIENTED_EDGE('',*,*,#6493,.F.);
#8514=ORIENTED_EDGE('',*,*,#6494,.T.);
#8515=ORIENTED_EDGE('',*,*,#6495,.F.);
#8516=ORIENTED_EDGE('',*,*,#6490,.F.);
#8517=ORIENTED_EDGE('',*,*,#6496,.F.);
#8518=ORIENTED_EDGE('',*,*,#6497,.T.);
#8519=ORIENTED_EDGE('',*,*,#6498,.F.);
#8520=ORIENTED_EDGE('',*,*,#6494,.F.);
#8521=ORIENTED_EDGE('',*,*,#6499,.F.);
#8522=ORIENTED_EDGE('',*,*,#6500,.T.);
#8523=ORIENTED_EDGE('',*,*,#6501,.F.);
#8524=ORIENTED_EDGE('',*,*,#6497,.F.);
#8525=ORIENTED_EDGE('',*,*,#6502,.F.);
#8526=ORIENTED_EDGE('',*,*,#6503,.T.);
#8527=ORIENTED_EDGE('',*,*,#6504,.F.);
#8528=ORIENTED_EDGE('',*,*,#6500,.F.);
#8529=ORIENTED_EDGE('',*,*,#6505,.F.);
#8530=ORIENTED_EDGE('',*,*,#6506,.T.);
#8531=ORIENTED_EDGE('',*,*,#6507,.F.);
#8532=ORIENTED_EDGE('',*,*,#6503,.F.);
#8533=ORIENTED_EDGE('',*,*,#6508,.F.);
#8534=ORIENTED_EDGE('',*,*,#6509,.T.);
#8535=ORIENTED_EDGE('',*,*,#6510,.F.);
#8536=ORIENTED_EDGE('',*,*,#6506,.F.);
#8537=ORIENTED_EDGE('',*,*,#6511,.F.);
#8538=ORIENTED_EDGE('',*,*,#6512,.T.);
#8539=ORIENTED_EDGE('',*,*,#6513,.F.);
#8540=ORIENTED_EDGE('',*,*,#6509,.F.);
#8541=ORIENTED_EDGE('',*,*,#6514,.F.);
#8542=ORIENTED_EDGE('',*,*,#6515,.F.);
#8543=ORIENTED_EDGE('',*,*,#6516,.F.);
#8544=ORIENTED_EDGE('',*,*,#6512,.F.);
#8545=ORIENTED_EDGE('',*,*,#6517,.F.);
#8546=ORIENTED_EDGE('',*,*,#6518,.T.);
#8547=ORIENTED_EDGE('',*,*,#6519,.F.);
#8548=ORIENTED_EDGE('',*,*,#6520,.F.);
#8549=ORIENTED_EDGE('',*,*,#6521,.F.);
#8550=ORIENTED_EDGE('',*,*,#6522,.T.);
#8551=ORIENTED_EDGE('',*,*,#6523,.F.);
#8552=ORIENTED_EDGE('',*,*,#6518,.F.);
#8553=ORIENTED_EDGE('',*,*,#6524,.F.);
#8554=ORIENTED_EDGE('',*,*,#6525,.T.);
#8555=ORIENTED_EDGE('',*,*,#6526,.F.);
#8556=ORIENTED_EDGE('',*,*,#6522,.F.);
#8557=ORIENTED_EDGE('',*,*,#6527,.F.);
#8558=ORIENTED_EDGE('',*,*,#6528,.T.);
#8559=ORIENTED_EDGE('',*,*,#6529,.F.);
#8560=ORIENTED_EDGE('',*,*,#6525,.F.);
#8561=ORIENTED_EDGE('',*,*,#6530,.F.);
#8562=ORIENTED_EDGE('',*,*,#6531,.T.);
#8563=ORIENTED_EDGE('',*,*,#6532,.F.);
#8564=ORIENTED_EDGE('',*,*,#6528,.F.);
#8565=ORIENTED_EDGE('',*,*,#6533,.F.);
#8566=ORIENTED_EDGE('',*,*,#6534,.T.);
#8567=ORIENTED_EDGE('',*,*,#6535,.F.);
#8568=ORIENTED_EDGE('',*,*,#6531,.F.);
#8569=ORIENTED_EDGE('',*,*,#6536,.F.);
#8570=ORIENTED_EDGE('',*,*,#6537,.T.);
#8571=ORIENTED_EDGE('',*,*,#6538,.F.);
#8572=ORIENTED_EDGE('',*,*,#6534,.F.);
#8573=ORIENTED_EDGE('',*,*,#6539,.F.);
#8574=ORIENTED_EDGE('',*,*,#6540,.T.);
#8575=ORIENTED_EDGE('',*,*,#6541,.F.);
#8576=ORIENTED_EDGE('',*,*,#6537,.F.);
#8577=ORIENTED_EDGE('',*,*,#6542,.F.);
#8578=ORIENTED_EDGE('',*,*,#6543,.F.);
#8579=ORIENTED_EDGE('',*,*,#6544,.F.);
#8580=ORIENTED_EDGE('',*,*,#6540,.F.);
#8581=ORIENTED_EDGE('',*,*,#6545,.F.);
#8582=ORIENTED_EDGE('',*,*,#6546,.T.);
#8583=ORIENTED_EDGE('',*,*,#6547,.F.);
#8584=ORIENTED_EDGE('',*,*,#6546,.F.);
#8585=ORIENTED_EDGE('',*,*,#6459,.T.);
#8586=ORIENTED_EDGE('',*,*,#6548,.T.);
#8587=ORIENTED_EDGE('',*,*,#6549,.T.);
#8588=ORIENTED_EDGE('',*,*,#6550,.F.);
#8589=ORIENTED_EDGE('',*,*,#6436,.T.);
#8590=ORIENTED_EDGE('',*,*,#6551,.F.);
#8591=ORIENTED_EDGE('',*,*,#6552,.F.);
#8592=ORIENTED_EDGE('',*,*,#6553,.T.);
#8593=ORIENTED_EDGE('',*,*,#6487,.T.);
#8594=ORIENTED_EDGE('',*,*,#6554,.T.);
#8595=ORIENTED_EDGE('',*,*,#6552,.T.);
#8596=ORIENTED_EDGE('',*,*,#6555,.F.);
#8597=ORIENTED_EDGE('',*,*,#6464,.T.);
#8598=ORIENTED_EDGE('',*,*,#6556,.F.);
#8599=ORIENTED_EDGE('',*,*,#6557,.F.);
#8600=ORIENTED_EDGE('',*,*,#6558,.T.);
#8601=ORIENTED_EDGE('',*,*,#6515,.T.);
#8602=ORIENTED_EDGE('',*,*,#6559,.T.);
#8603=ORIENTED_EDGE('',*,*,#6557,.T.);
#8604=ORIENTED_EDGE('',*,*,#6560,.F.);
#8605=ORIENTED_EDGE('',*,*,#6492,.T.);
#8606=ORIENTED_EDGE('',*,*,#6561,.F.);
#8607=ORIENTED_EDGE('',*,*,#6562,.F.);
#8608=ORIENTED_EDGE('',*,*,#6563,.T.);
#8609=ORIENTED_EDGE('',*,*,#6543,.T.);
#8610=ORIENTED_EDGE('',*,*,#6564,.T.);
#8611=ORIENTED_EDGE('',*,*,#6562,.T.);
#8612=ORIENTED_EDGE('',*,*,#6565,.F.);
#8613=ORIENTED_EDGE('',*,*,#6520,.T.);
#8614=ORIENTED_EDGE('',*,*,#6566,.F.);
#8615=ORIENTED_EDGE('',*,*,#6549,.F.);
#8616=ORIENTED_EDGE('',*,*,#6567,.T.);
#8617=ORIENTED_EDGE('',*,*,#6435,.T.);
#8618=ORIENTED_EDGE('',*,*,#6439,.T.);
#8619=ORIENTED_EDGE('',*,*,#6442,.T.);
#8620=ORIENTED_EDGE('',*,*,#6445,.T.);
#8621=ORIENTED_EDGE('',*,*,#6448,.T.);
#8622=ORIENTED_EDGE('',*,*,#6451,.T.);
#8623=ORIENTED_EDGE('',*,*,#6454,.T.);
#8624=ORIENTED_EDGE('',*,*,#6457,.T.);
#8625=ORIENTED_EDGE('',*,*,#6460,.T.);
#8626=ORIENTED_EDGE('',*,*,#6550,.T.);
#8627=ORIENTED_EDGE('',*,*,#6566,.T.);
#8628=ORIENTED_EDGE('',*,*,#6519,.T.);
#8629=ORIENTED_EDGE('',*,*,#6523,.T.);
#8630=ORIENTED_EDGE('',*,*,#6526,.T.);
#8631=ORIENTED_EDGE('',*,*,#6529,.T.);
#8632=ORIENTED_EDGE('',*,*,#6532,.T.);
#8633=ORIENTED_EDGE('',*,*,#6535,.T.);
#8634=ORIENTED_EDGE('',*,*,#6538,.T.);
#8635=ORIENTED_EDGE('',*,*,#6541,.T.);
#8636=ORIENTED_EDGE('',*,*,#6544,.T.);
#8637=ORIENTED_EDGE('',*,*,#6565,.T.);
#8638=ORIENTED_EDGE('',*,*,#6561,.T.);
#8639=ORIENTED_EDGE('',*,*,#6491,.T.);
#8640=ORIENTED_EDGE('',*,*,#6495,.T.);
#8641=ORIENTED_EDGE('',*,*,#6498,.T.);
#8642=ORIENTED_EDGE('',*,*,#6501,.T.);
#8643=ORIENTED_EDGE('',*,*,#6504,.T.);
#8644=ORIENTED_EDGE('',*,*,#6507,.T.);
#8645=ORIENTED_EDGE('',*,*,#6510,.T.);
#8646=ORIENTED_EDGE('',*,*,#6513,.T.);
#8647=ORIENTED_EDGE('',*,*,#6516,.T.);
#8648=ORIENTED_EDGE('',*,*,#6560,.T.);
#8649=ORIENTED_EDGE('',*,*,#6556,.T.);
#8650=ORIENTED_EDGE('',*,*,#6463,.T.);
#8651=ORIENTED_EDGE('',*,*,#6467,.T.);
#8652=ORIENTED_EDGE('',*,*,#6470,.T.);
#8653=ORIENTED_EDGE('',*,*,#6473,.T.);
#8654=ORIENTED_EDGE('',*,*,#6476,.T.);
#8655=ORIENTED_EDGE('',*,*,#6479,.T.);
#8656=ORIENTED_EDGE('',*,*,#6482,.T.);
#8657=ORIENTED_EDGE('',*,*,#6485,.T.);
#8658=ORIENTED_EDGE('',*,*,#6488,.T.);
#8659=ORIENTED_EDGE('',*,*,#6555,.T.);
#8660=ORIENTED_EDGE('',*,*,#6551,.T.);
#8661=ORIENTED_EDGE('',*,*,#6547,.T.);
#8662=ORIENTED_EDGE('',*,*,#6433,.T.);
#8663=ORIENTED_EDGE('',*,*,#6553,.F.);
#8664=ORIENTED_EDGE('',*,*,#6554,.F.);
#8665=ORIENTED_EDGE('',*,*,#6486,.T.);
#8666=ORIENTED_EDGE('',*,*,#6483,.T.);
#8667=ORIENTED_EDGE('',*,*,#6480,.T.);
#8668=ORIENTED_EDGE('',*,*,#6477,.T.);
#8669=ORIENTED_EDGE('',*,*,#6474,.T.);
#8670=ORIENTED_EDGE('',*,*,#6471,.T.);
#8671=ORIENTED_EDGE('',*,*,#6468,.T.);
#8672=ORIENTED_EDGE('',*,*,#6465,.T.);
#8673=ORIENTED_EDGE('',*,*,#6461,.T.);
#8674=ORIENTED_EDGE('',*,*,#6558,.F.);
#8675=ORIENTED_EDGE('',*,*,#6559,.F.);
#8676=ORIENTED_EDGE('',*,*,#6514,.T.);
#8677=ORIENTED_EDGE('',*,*,#6511,.T.);
#8678=ORIENTED_EDGE('',*,*,#6508,.T.);
#8679=ORIENTED_EDGE('',*,*,#6505,.T.);
#8680=ORIENTED_EDGE('',*,*,#6502,.T.);
#8681=ORIENTED_EDGE('',*,*,#6499,.T.);
#8682=ORIENTED_EDGE('',*,*,#6496,.T.);
#8683=ORIENTED_EDGE('',*,*,#6493,.T.);
#8684=ORIENTED_EDGE('',*,*,#6489,.T.);
#8685=ORIENTED_EDGE('',*,*,#6563,.F.);
#8686=ORIENTED_EDGE('',*,*,#6564,.F.);
#8687=ORIENTED_EDGE('',*,*,#6542,.T.);
#8688=ORIENTED_EDGE('',*,*,#6539,.T.);
#8689=ORIENTED_EDGE('',*,*,#6536,.T.);
#8690=ORIENTED_EDGE('',*,*,#6533,.T.);
#8691=ORIENTED_EDGE('',*,*,#6530,.T.);
#8692=ORIENTED_EDGE('',*,*,#6527,.T.);
#8693=ORIENTED_EDGE('',*,*,#6524,.T.);
#8694=ORIENTED_EDGE('',*,*,#6521,.T.);
#8695=ORIENTED_EDGE('',*,*,#6517,.T.);
#8696=ORIENTED_EDGE('',*,*,#6567,.F.);
#8697=ORIENTED_EDGE('',*,*,#6548,.F.);
#8698=ORIENTED_EDGE('',*,*,#6458,.T.);
#8699=ORIENTED_EDGE('',*,*,#6455,.T.);
#8700=ORIENTED_EDGE('',*,*,#6452,.T.);
#8701=ORIENTED_EDGE('',*,*,#6449,.T.);
#8702=ORIENTED_EDGE('',*,*,#6446,.T.);
#8703=ORIENTED_EDGE('',*,*,#6443,.T.);
#8704=ORIENTED_EDGE('',*,*,#6440,.T.);
#8705=ORIENTED_EDGE('',*,*,#6437,.T.);
#8706=ORIENTED_EDGE('',*,*,#6545,.T.);
#10187=CYLINDRICAL_SURFACE('',#12087,0.21);
#10566=ADVANCED_FACE('',(#1515),#1022,.F.);
#10567=ADVANCED_FACE('',(#1516),#1023,.F.);
#10568=ADVANCED_FACE('',(#1517),#1024,.F.);
#10569=ADVANCED_FACE('',(#1518),#1025,.F.);
#10570=ADVANCED_FACE('',(#1519),#1026,.F.);
#10571=ADVANCED_FACE('',(#1520),#1027,.F.);
#10572=ADVANCED_FACE('',(#1521),#1028,.F.);
#10573=ADVANCED_FACE('',(#1522),#1029,.F.);
#10574=ADVANCED_FACE('',(#1523),#1030,.F.);
#10575=ADVANCED_FACE('',(#1524),#1031,.F.);
#10576=ADVANCED_FACE('',(#1525),#1032,.F.);
#10577=ADVANCED_FACE('',(#1526),#1033,.F.);
#10578=ADVANCED_FACE('',(#1527),#1034,.F.);
#10579=ADVANCED_FACE('',(#1528),#1035,.F.);
#10580=ADVANCED_FACE('',(#1529),#1036,.F.);
#10581=ADVANCED_FACE('',(#1530),#1037,.F.);
#10582=ADVANCED_FACE('',(#1531),#1038,.F.);
#10583=ADVANCED_FACE('',(#1532),#1039,.F.);
#10584=ADVANCED_FACE('',(#1533),#1040,.F.);
#10585=ADVANCED_FACE('',(#1534),#1041,.F.);
#10586=ADVANCED_FACE('',(#1535),#1042,.F.);
#10587=ADVANCED_FACE('',(#1536),#1043,.F.);
#10588=ADVANCED_FACE('',(#1537),#1044,.F.);
#10589=ADVANCED_FACE('',(#1538),#1045,.F.);
#10590=ADVANCED_FACE('',(#1539),#1046,.F.);
#10591=ADVANCED_FACE('',(#1540),#1047,.F.);
#10592=ADVANCED_FACE('',(#1541),#1048,.F.);
#10593=ADVANCED_FACE('',(#1542),#1049,.F.);
#10594=ADVANCED_FACE('',(#1543),#1050,.F.);
#10595=ADVANCED_FACE('',(#1544),#1051,.F.);
#10596=ADVANCED_FACE('',(#1545),#1052,.F.);
#10597=ADVANCED_FACE('',(#1546),#1053,.F.);
#10598=ADVANCED_FACE('',(#1547),#1054,.F.);
#10599=ADVANCED_FACE('',(#1548),#1055,.F.);
#10600=ADVANCED_FACE('',(#1549),#1056,.F.);
#10601=ADVANCED_FACE('',(#1550),#1057,.F.);
#10602=ADVANCED_FACE('',(#1551),#10187,.F.);
#10603=ADVANCED_FACE('',(#1552),#1058,.T.);
#10604=ADVANCED_FACE('',(#1553),#1059,.T.);
#10605=ADVANCED_FACE('',(#1554),#1060,.T.);
#10606=ADVANCED_FACE('',(#1555),#1061,.T.);
#10607=ADVANCED_FACE('',(#1556),#1062,.T.);
#10608=ADVANCED_FACE('',(#1557),#1063,.T.);
#10609=ADVANCED_FACE('',(#1558),#1064,.T.);
#10610=ADVANCED_FACE('',(#1559),#1065,.T.);
#10611=ADVANCED_FACE('',(#1560,#813),#1066,.T.);
#10612=ADVANCED_FACE('',(#1561,#814),#1067,.F.);
#10952=CLOSED_SHELL('',(#10566,#10567,#10568,#10569,#10570,#10571,#10572,
#10573,#10574,#10575,#10576,#10577,#10578,#10579,#10580,#10581,#10582,#10583,
#10584,#10585,#10586,#10587,#10588,#10589,#10590,#10591,#10592,#10593,#10594,
#10595,#10596,#10597,#10598,#10599,#10600,#10601,#10602,#10603,#10604,#10605,
#10606,#10607,#10608,#10609,#10610,#10611,#10612));
#12050=AXIS2_PLACEMENT_3D('',#17858,#14211,#14212);
#12051=AXIS2_PLACEMENT_3D('',#17859,#14213,#14214);
#12052=AXIS2_PLACEMENT_3D('',#17868,#14219,#14220);
#12053=AXIS2_PLACEMENT_3D('',#17874,#14224,#14225);
#12054=AXIS2_PLACEMENT_3D('',#17880,#14229,#14230);
#12055=AXIS2_PLACEMENT_3D('',#17886,#14234,#14235);
#12056=AXIS2_PLACEMENT_3D('',#17892,#14239,#14240);
#12057=AXIS2_PLACEMENT_3D('',#17898,#14244,#14245);
#12058=AXIS2_PLACEMENT_3D('',#17904,#14249,#14250);
#12059=AXIS2_PLACEMENT_3D('',#17910,#14254,#14255);
#12060=AXIS2_PLACEMENT_3D('',#17916,#14259,#14260);
#12061=AXIS2_PLACEMENT_3D('',#17925,#14265,#14266);
#12062=AXIS2_PLACEMENT_3D('',#17931,#14270,#14271);
#12063=AXIS2_PLACEMENT_3D('',#17937,#14275,#14276);
#12064=AXIS2_PLACEMENT_3D('',#17943,#14280,#14281);
#12065=AXIS2_PLACEMENT_3D('',#17949,#14285,#14286);
#12066=AXIS2_PLACEMENT_3D('',#17955,#14290,#14291);
#12067=AXIS2_PLACEMENT_3D('',#17961,#14295,#14296);
#12068=AXIS2_PLACEMENT_3D('',#17967,#14300,#14301);
#12069=AXIS2_PLACEMENT_3D('',#17973,#14305,#14306);
#12070=AXIS2_PLACEMENT_3D('',#17982,#14311,#14312);
#12071=AXIS2_PLACEMENT_3D('',#17988,#14316,#14317);
#12072=AXIS2_PLACEMENT_3D('',#17994,#14321,#14322);
#12073=AXIS2_PLACEMENT_3D('',#18000,#14326,#14327);
#12074=AXIS2_PLACEMENT_3D('',#18006,#14331,#14332);
#12075=AXIS2_PLACEMENT_3D('',#18012,#14336,#14337);
#12076=AXIS2_PLACEMENT_3D('',#18018,#14341,#14342);
#12077=AXIS2_PLACEMENT_3D('',#18024,#14346,#14347);
#12078=AXIS2_PLACEMENT_3D('',#18030,#14351,#14352);
#12079=AXIS2_PLACEMENT_3D('',#18039,#14357,#14358);
#12080=AXIS2_PLACEMENT_3D('',#18045,#14362,#14363);
#12081=AXIS2_PLACEMENT_3D('',#18051,#14367,#14368);
#12082=AXIS2_PLACEMENT_3D('',#18057,#14372,#14373);
#12083=AXIS2_PLACEMENT_3D('',#18063,#14377,#14378);
#12084=AXIS2_PLACEMENT_3D('',#18069,#14382,#14383);
#12085=AXIS2_PLACEMENT_3D('',#18075,#14387,#14388);
#12086=AXIS2_PLACEMENT_3D('',#18081,#14392,#14393);
#12087=AXIS2_PLACEMENT_3D('',#18087,#14397,#14398);
#12088=AXIS2_PLACEMENT_3D('',#18089,#14399,#14400);
#12089=AXIS2_PLACEMENT_3D('',#18092,#14402,#14403);
#12090=AXIS2_PLACEMENT_3D('',#18093,#14404,#14405);
#12091=AXIS2_PLACEMENT_3D('',#18099,#14409,#14410);
#12092=AXIS2_PLACEMENT_3D('',#18105,#14414,#14415);
#12093=AXIS2_PLACEMENT_3D('',#18108,#14418,#14419);
#12094=AXIS2_PLACEMENT_3D('',#18114,#14423,#14424);
#12095=AXIS2_PLACEMENT_3D('',#18117,#14427,#14428);
#12096=AXIS2_PLACEMENT_3D('',#18123,#14432,#14433);
#12097=AXIS2_PLACEMENT_3D('',#18126,#14436,#14437);
#12098=AXIS2_PLACEMENT_3D('',#18129,#14440,#14441);
#12099=AXIS2_PLACEMENT_3D('',#18130,#14442,#14443);
#14211=DIRECTION('axis',(0.,0.,1.));
#14212=DIRECTION('refdir',(1.,0.,0.));
#14213=DIRECTION('center_axis',(0.,0.,-1.));
#14214=DIRECTION('ref_axis',(0.,1.,0.));
#14215=DIRECTION('',(0.,1.,0.));
#14216=DIRECTION('',(1.,0.,0.));
#14217=DIRECTION('',(0.,-1.,0.));
#14218=DIRECTION('',(1.,0.,0.));
#14219=DIRECTION('center_axis',(0.,1.,-8.88178419700125E-16));
#14220=DIRECTION('ref_axis',(0.,8.88178419700125E-16,1.));
#14221=DIRECTION('',(0.,8.88178419700125E-16,1.));
#14222=DIRECTION('',(1.,0.,0.));
#14223=DIRECTION('',(0.,-8.88178419700125E-16,-1.));
#14224=DIRECTION('center_axis',(0.,-7.40148683083439E-16,-1.));
#14225=DIRECTION('ref_axis',(0.,1.,-7.40148683083439E-16));
#14226=DIRECTION('',(0.,1.,-7.40148683083439E-16));
#14227=DIRECTION('',(1.,0.,0.));
#14228=DIRECTION('',(0.,-1.,7.40148683083439E-16));
#14229=DIRECTION('center_axis',(0.,-0.707106781186547,-0.707106781186548));
#14230=DIRECTION('ref_axis',(0.,0.707106781186548,-0.707106781186547));
#14231=DIRECTION('',(0.,0.707106781186548,-0.707106781186547));
#14232=DIRECTION('',(1.,0.,0.));
#14233=DIRECTION('',(0.,-0.707106781186548,0.707106781186547));
#14234=DIRECTION('center_axis',(0.,-1.,2.77555756156289E-16));
#14235=DIRECTION('ref_axis',(0.,-2.77555756156289E-16,-1.));
#14236=DIRECTION('',(0.,-2.77555756156289E-16,-1.));
#14237=DIRECTION('',(1.,0.,0.));
#14238=DIRECTION('',(0.,2.77555756156289E-16,1.));
#14239=DIRECTION('center_axis',(0.,-0.707106781186547,0.707106781186548));
#14240=DIRECTION('ref_axis',(0.,-0.707106781186548,-0.707106781186547));
#14241=DIRECTION('',(0.,-0.707106781186548,-0.707106781186547));
#14242=DIRECTION('',(1.,0.,0.));
#14243=DIRECTION('',(0.,0.707106781186548,0.707106781186547));
#14244=DIRECTION('center_axis',(0.,7.40148683083438E-16,1.));
#14245=DIRECTION('ref_axis',(0.,-1.,7.40148683083438E-16));
#14246=DIRECTION('',(0.,-1.,7.40148683083438E-16));
#14247=DIRECTION('',(1.,0.,0.));
#14248=DIRECTION('',(0.,1.,-7.40148683083438E-16));
#14249=DIRECTION('center_axis',(0.,1.,-4.44089209850063E-16));
#14250=DIRECTION('ref_axis',(0.,4.44089209850063E-16,1.));
#14251=DIRECTION('',(0.,4.44089209850063E-16,1.));
#14252=DIRECTION('',(1.,0.,0.));
#14253=DIRECTION('',(0.,-4.44089209850063E-16,-1.));
#14254=DIRECTION('center_axis',(0.,2.41352831440251E-16,1.));
#14255=DIRECTION('ref_axis',(0.,-1.,2.41352831440251E-16));
#14256=DIRECTION('',(0.,-1.,2.41352831440251E-16));
#14257=DIRECTION('',(-1.,0.,0.));
#14258=DIRECTION('',(0.,1.,-2.41352831440251E-16));
#14259=DIRECTION('center_axis',(0.,-1.,2.41352831440251E-16));
#14260=DIRECTION('ref_axis',(0.,-2.41352831440251E-16,-1.));
#14261=DIRECTION('',(0.,-2.41352831440251E-16,-1.));
#14262=DIRECTION('',(1.,0.,0.));
#14263=DIRECTION('',(0.,2.41352831440251E-16,1.));
#14264=DIRECTION('',(1.,0.,0.));
#14265=DIRECTION('center_axis',(0.,0.,-1.));
#14266=DIRECTION('ref_axis',(0.,1.,0.));
#14267=DIRECTION('',(0.,1.,0.));
#14268=DIRECTION('',(1.,0.,0.));
#14269=DIRECTION('',(0.,-1.,0.));
#14270=DIRECTION('center_axis',(0.,-1.,0.));
#14271=DIRECTION('ref_axis',(0.,0.,-1.));
#14272=DIRECTION('',(0.,0.,-1.));
#14273=DIRECTION('',(1.,0.,0.));
#14274=DIRECTION('',(0.,0.,1.));
#14275=DIRECTION('center_axis',(0.,-0.707106781186547,0.707106781186548));
#14276=DIRECTION('ref_axis',(0.,-0.707106781186548,-0.707106781186547));
#14277=DIRECTION('',(0.,-0.707106781186548,-0.707106781186547));
#14278=DIRECTION('',(1.,0.,0.));
#14279=DIRECTION('',(0.,0.707106781186548,0.707106781186547));
#14280=DIRECTION('center_axis',(0.,0.,1.));
#14281=DIRECTION('ref_axis',(0.,-1.,0.));
#14282=DIRECTION('',(0.,-1.,0.));
#14283=DIRECTION('',(1.,0.,0.));
#14284=DIRECTION('',(0.,1.,0.));
#14285=DIRECTION('center_axis',(0.,0.707106781186548,0.707106781186547));
#14286=DIRECTION('ref_axis',(0.,-0.707106781186547,0.707106781186548));
#14287=DIRECTION('',(0.,-0.707106781186547,0.707106781186548));
#14288=DIRECTION('',(1.,0.,0.));
#14289=DIRECTION('',(0.,0.707106781186547,-0.707106781186548));
#14290=DIRECTION('center_axis',(0.,1.,0.));
#14291=DIRECTION('ref_axis',(0.,0.,1.));
#14292=DIRECTION('',(0.,0.,1.));
#14293=DIRECTION('',(1.,0.,0.));
#14294=DIRECTION('',(0.,0.,-1.));
#14295=DIRECTION('center_axis',(0.,0.,-1.));
#14296=DIRECTION('ref_axis',(0.,1.,0.));
#14297=DIRECTION('',(0.,1.,0.));
#14298=DIRECTION('',(1.,0.,0.));
#14299=DIRECTION('',(0.,-1.,0.));
#14300=DIRECTION('center_axis',(0.,1.,-2.41352831440251E-16));
#14301=DIRECTION('ref_axis',(0.,2.41352831440251E-16,1.));
#14302=DIRECTION('',(0.,2.41352831440251E-16,1.));
#14303=DIRECTION('',(-1.,0.,0.));
#14304=DIRECTION('',(0.,-2.41352831440251E-16,-1.));
#14305=DIRECTION('center_axis',(0.,0.,1.));
#14306=DIRECTION('ref_axis',(0.,-1.,0.));
#14307=DIRECTION('',(0.,-1.,0.));
#14308=DIRECTION('',(1.,0.,0.));
#14309=DIRECTION('',(0.,1.,0.));
#14310=DIRECTION('',(1.,0.,0.));
#14311=DIRECTION('center_axis',(0.,-1.,0.));
#14312=DIRECTION('ref_axis',(0.,0.,-1.));
#14313=DIRECTION('',(0.,0.,-1.));
#14314=DIRECTION('',(1.,0.,0.));
#14315=DIRECTION('',(0.,0.,1.));
#14316=DIRECTION('center_axis',(0.,0.,1.));
#14317=DIRECTION('ref_axis',(0.,-1.,0.));
#14318=DIRECTION('',(0.,-1.,0.));
#14319=DIRECTION('',(1.,0.,0.));
#14320=DIRECTION('',(0.,1.,0.));
#14321=DIRECTION('center_axis',(0.,0.707106781186548,0.707106781186548));
#14322=DIRECTION('ref_axis',(0.,-0.707106781186548,0.707106781186548));
#14323=DIRECTION('',(0.,-0.707106781186548,0.707106781186548));
#14324=DIRECTION('',(1.,0.,0.));
#14325=DIRECTION('',(0.,0.707106781186548,-0.707106781186548));
#14326=DIRECTION('center_axis',(0.,1.,0.));
#14327=DIRECTION('ref_axis',(0.,0.,1.));
#14328=DIRECTION('',(0.,0.,1.));
#14329=DIRECTION('',(1.,0.,0.));
#14330=DIRECTION('',(0.,0.,-1.));
#14331=DIRECTION('center_axis',(0.,0.707106781186548,-0.707106781186547));
#14332=DIRECTION('ref_axis',(0.,0.707106781186547,0.707106781186548));
#14333=DIRECTION('',(0.,0.707106781186547,0.707106781186548));
#14334=DIRECTION('',(1.,0.,0.));
#14335=DIRECTION('',(0.,-0.707106781186547,-0.707106781186548));
#14336=DIRECTION('center_axis',(0.,-7.40148683083438E-16,-1.));
#14337=DIRECTION('ref_axis',(0.,1.,-7.40148683083438E-16));
#14338=DIRECTION('',(0.,1.,-7.40148683083438E-16));
#14339=DIRECTION('',(1.,0.,0.));
#14340=DIRECTION('',(0.,-1.,7.40148683083438E-16));
#14341=DIRECTION('center_axis',(0.,-1.,0.));
#14342=DIRECTION('ref_axis',(0.,0.,-1.));
#14343=DIRECTION('',(0.,0.,-1.));
#14344=DIRECTION('',(1.,0.,0.));
#14345=DIRECTION('',(0.,0.,1.));
#14346=DIRECTION('center_axis',(0.,0.,-1.));
#14347=DIRECTION('ref_axis',(0.,1.,0.));
#14348=DIRECTION('',(0.,1.,0.));
#14349=DIRECTION('',(-1.,0.,0.));
#14350=DIRECTION('',(0.,-1.,0.));
#14351=DIRECTION('center_axis',(0.,1.,0.));
#14352=DIRECTION('ref_axis',(0.,0.,1.));
#14353=DIRECTION('',(0.,0.,1.));
#14354=DIRECTION('',(1.,0.,0.));
#14355=DIRECTION('',(0.,0.,-1.));
#14356=DIRECTION('',(1.,0.,0.));
#14357=DIRECTION('center_axis',(0.,0.,1.));
#14358=DIRECTION('ref_axis',(0.,-1.,0.));
#14359=DIRECTION('',(0.,-1.,0.));
#14360=DIRECTION('',(1.,0.,0.));
#14361=DIRECTION('',(0.,1.,0.));
#14362=DIRECTION('center_axis',(0.,1.,0.));
#14363=DIRECTION('ref_axis',(0.,0.,1.));
#14364=DIRECTION('',(0.,0.,1.));
#14365=DIRECTION('',(1.,0.,0.));
#14366=DIRECTION('',(0.,0.,-1.));
#14367=DIRECTION('center_axis',(0.,0.707106781186547,-0.707106781186548));
#14368=DIRECTION('ref_axis',(0.,0.707106781186548,0.707106781186547));
#14369=DIRECTION('',(0.,0.707106781186548,0.707106781186547));
#14370=DIRECTION('',(1.,0.,0.));
#14371=DIRECTION('',(0.,-0.707106781186548,-0.707106781186547));
#14372=DIRECTION('center_axis',(0.,0.,-1.));
#14373=DIRECTION('ref_axis',(0.,1.,0.));
#14374=DIRECTION('',(0.,1.,0.));
#14375=DIRECTION('',(1.,0.,0.));
#14376=DIRECTION('',(0.,-1.,0.));
#14377=DIRECTION('center_axis',(0.,-0.707106781186547,-0.707106781186548));
#14378=DIRECTION('ref_axis',(0.,0.707106781186548,-0.707106781186547));
#14379=DIRECTION('',(0.,0.707106781186548,-0.707106781186547));
#14380=DIRECTION('',(1.,0.,0.));
#14381=DIRECTION('',(0.,-0.707106781186548,0.707106781186547));
#14382=DIRECTION('center_axis',(0.,-1.,0.));
#14383=DIRECTION('ref_axis',(0.,0.,-1.));
#14384=DIRECTION('',(0.,0.,-1.));
#14385=DIRECTION('',(1.,0.,0.));
#14386=DIRECTION('',(0.,0.,1.));
#14387=DIRECTION('center_axis',(0.,0.,1.));
#14388=DIRECTION('ref_axis',(0.,-1.,0.));
#14389=DIRECTION('',(0.,-1.,0.));
#14390=DIRECTION('',(1.,0.,0.));
#14391=DIRECTION('',(0.,1.,0.));
#14392=DIRECTION('center_axis',(0.,-1.,0.));
#14393=DIRECTION('ref_axis',(0.,0.,-1.));
#14394=DIRECTION('',(0.,0.,-1.));
#14395=DIRECTION('',(-1.,0.,0.));
#14396=DIRECTION('',(0.,0.,1.));
#14397=DIRECTION('center_axis',(1.,0.,0.));
#14398=DIRECTION('ref_axis',(0.,0.,-1.));
#14399=DIRECTION('center_axis',(1.,0.,0.));
#14400=DIRECTION('ref_axis',(0.,0.,-1.));
#14401=DIRECTION('',(1.,0.,0.));
#14402=DIRECTION('center_axis',(-1.,0.,0.));
#14403=DIRECTION('ref_axis',(0.,0.,-1.));
#14404=DIRECTION('center_axis',(0.,1.,0.));
#14405=DIRECTION('ref_axis',(0.,0.,1.));
#14406=DIRECTION('',(0.,0.,1.));
#14407=DIRECTION('',(1.,0.,0.));
#14408=DIRECTION('',(0.,0.,1.));
#14409=DIRECTION('center_axis',(0.,1.,0.));
#14410=DIRECTION('ref_axis',(0.,0.,1.));
#14411=DIRECTION('',(0.,0.,1.));
#14412=DIRECTION('',(1.,0.,0.));
#14413=DIRECTION('',(0.,0.,1.));
#14414=DIRECTION('center_axis',(0.,0.,-1.));
#14415=DIRECTION('ref_axis',(0.,1.,0.));
#14416=DIRECTION('',(0.,1.,0.));
#14417=DIRECTION('',(0.,1.,0.));
#14418=DIRECTION('center_axis',(0.,0.,-1.));
#14419=DIRECTION('ref_axis',(0.,1.,0.));
#14420=DIRECTION('',(0.,1.,0.));
#14421=DIRECTION('',(1.,0.,0.));
#14422=DIRECTION('',(0.,1.,0.));
#14423=DIRECTION('center_axis',(0.,-1.,0.));
#14424=DIRECTION('ref_axis',(0.,0.,-1.));
#14425=DIRECTION('',(0.,0.,-1.));
#14426=DIRECTION('',(0.,0.,-1.));
#14427=DIRECTION('center_axis',(0.,-1.,0.));
#14428=DIRECTION('ref_axis',(0.,0.,-1.));
#14429=DIRECTION('',(0.,0.,-1.));
#14430=DIRECTION('',(1.,0.,0.));
#14431=DIRECTION('',(0.,0.,-1.));
#14432=DIRECTION('center_axis',(0.,0.,1.));
#14433=DIRECTION('ref_axis',(0.,-1.,0.));
#14434=DIRECTION('',(0.,-1.,0.));
#14435=DIRECTION('',(0.,-1.,0.));
#14436=DIRECTION('center_axis',(0.,0.,1.));
#14437=DIRECTION('ref_axis',(0.,-1.,0.));
#14438=DIRECTION('',(0.,-1.,0.));
#14439=DIRECTION('',(0.,-1.,0.));
#14440=DIRECTION('center_axis',(1.,0.,0.));
#14441=DIRECTION('ref_axis',(0.,0.,-1.));
#14442=DIRECTION('center_axis',(1.,0.,0.));
#14443=DIRECTION('ref_axis',(0.,0.,-1.));
#17858=CARTESIAN_POINT('',(0.,0.,0.));
#17859=CARTESIAN_POINT('Origin',(-0.1,0.82,-0.3));
#17860=CARTESIAN_POINT('',(0.,0.82,-0.3));
#17861=CARTESIAN_POINT('',(0.,1.,-0.3));
#17862=CARTESIAN_POINT('',(0.,0.41,-0.3));
#17863=CARTESIAN_POINT('',(40.,0.82,-0.3));
#17864=CARTESIAN_POINT('',(-0.1,0.82,-0.3));
#17865=CARTESIAN_POINT('',(40.,1.,-0.3));
#17866=CARTESIAN_POINT('',(40.,0.41,-0.3));
#17867=CARTESIAN_POINT('',(-0.05,1.,-0.3));
#17868=CARTESIAN_POINT('Origin',(-0.1,0.82,-0.55));
#17869=CARTESIAN_POINT('',(0.,0.82,-0.55));
#17870=CARTESIAN_POINT('',(0.,0.82,-0.275));
#17871=CARTESIAN_POINT('',(40.,0.82,-0.55));
#17872=CARTESIAN_POINT('',(-0.1,0.82,-0.55));
#17873=CARTESIAN_POINT('',(40.,0.82,-0.275));
#17874=CARTESIAN_POINT('Origin',(-0.1,0.67,-0.55));
#17875=CARTESIAN_POINT('',(0.,0.67,-0.55));
#17876=CARTESIAN_POINT('',(0.,0.335,-0.55));
#17877=CARTESIAN_POINT('',(40.,0.67,-0.55));
#17878=CARTESIAN_POINT('',(-0.1,0.67,-0.55));
#17879=CARTESIAN_POINT('',(40.,0.335,-0.55));
#17880=CARTESIAN_POINT('Origin',(-0.1,0.42,-0.3));
#17881=CARTESIAN_POINT('',(0.,0.42,-0.3));
#17882=CARTESIAN_POINT('',(0.,0.24,-0.12));
#17883=CARTESIAN_POINT('',(40.,0.42,-0.3));
#17884=CARTESIAN_POINT('',(-0.1,0.42,-0.3));
#17885=CARTESIAN_POINT('',(40.,0.24,-0.12));
#17886=CARTESIAN_POINT('Origin',(-0.1,0.42,0.3));
#17887=CARTESIAN_POINT('',(0.,0.42,0.3));
#17888=CARTESIAN_POINT('',(0.,0.42,0.15));
#17889=CARTESIAN_POINT('',(40.,0.42,0.3));
#17890=CARTESIAN_POINT('',(-0.1,0.42,0.3));
#17891=CARTESIAN_POINT('',(40.,0.42,0.15));
#17892=CARTESIAN_POINT('Origin',(-0.1,0.67,0.55));
#17893=CARTESIAN_POINT('',(0.,0.67,0.55));
#17894=CARTESIAN_POINT('',(6.93889390390723E-18,0.365,0.245));
#17895=CARTESIAN_POINT('',(40.,0.67,0.55));
#17896=CARTESIAN_POINT('',(-0.1,0.67,0.55));
#17897=CARTESIAN_POINT('',(40.,0.365,0.245));
#17898=CARTESIAN_POINT('Origin',(-0.1,0.82,0.55));
#17899=CARTESIAN_POINT('',(0.,0.82,0.55));
#17900=CARTESIAN_POINT('',(0.,0.41,0.55));
#17901=CARTESIAN_POINT('',(40.,0.82,0.55));
#17902=CARTESIAN_POINT('',(-0.1,0.82,0.55));
#17903=CARTESIAN_POINT('',(40.,0.41,0.55));
#17904=CARTESIAN_POINT('Origin',(-0.1,0.82,0.3));
#17905=CARTESIAN_POINT('',(0.,0.82,0.3));
#17906=CARTESIAN_POINT('',(0.,0.82,0.15));
#17907=CARTESIAN_POINT('',(40.,0.82,0.3));
#17908=CARTESIAN_POINT('',(-0.1,0.82,0.3));
#17909=CARTESIAN_POINT('',(40.,0.82,0.15));
#17910=CARTESIAN_POINT('Origin',(-0.1,1.05,0.3));
#17911=CARTESIAN_POINT('',(0.,1.,0.3));
#17912=CARTESIAN_POINT('',(0.,0.525,0.3));
#17913=CARTESIAN_POINT('',(40.,1.,0.3));
#17914=CARTESIAN_POINT('',(-0.05,1.,0.3));
#17915=CARTESIAN_POINT('',(40.,0.525,0.3));
#17916=CARTESIAN_POINT('Origin',(-0.1,-0.3,-0.82));
#17917=CARTESIAN_POINT('',(0.,-0.3,-0.82));
#17918=CARTESIAN_POINT('',(0.,-0.3,-1.));
#17919=CARTESIAN_POINT('',(0.,-0.3,-0.41));
#17920=CARTESIAN_POINT('',(40.,-0.3,-0.82));
#17921=CARTESIAN_POINT('',(-0.1,-0.3,-0.82));
#17922=CARTESIAN_POINT('',(40.,-0.3,-1.));
#17923=CARTESIAN_POINT('',(40.,-0.3,-0.41));
#17924=CARTESIAN_POINT('',(-0.05,-0.3,-1.));
#17925=CARTESIAN_POINT('Origin',(-0.1,-0.55,-0.82));
#17926=CARTESIAN_POINT('',(0.,-0.55,-0.82));
#17927=CARTESIAN_POINT('',(0.,-0.275,-0.82));
#17928=CARTESIAN_POINT('',(40.,-0.55,-0.82));
#17929=CARTESIAN_POINT('',(-0.1,-0.55,-0.82));
#17930=CARTESIAN_POINT('',(40.,-0.275,-0.82));
#17931=CARTESIAN_POINT('Origin',(-0.1,-0.55,-0.67));
#17932=CARTESIAN_POINT('',(0.,-0.55,-0.67));
#17933=CARTESIAN_POINT('',(0.,-0.55,-0.335));
#17934=CARTESIAN_POINT('',(40.,-0.55,-0.67));
#17935=CARTESIAN_POINT('',(-0.1,-0.55,-0.67));
#17936=CARTESIAN_POINT('',(40.,-0.55,-0.335));
#17937=CARTESIAN_POINT('Origin',(-0.1,-0.3,-0.42));
#17938=CARTESIAN_POINT('',(0.,-0.3,-0.42));
#17939=CARTESIAN_POINT('',(0.,-0.12,-0.24));
#17940=CARTESIAN_POINT('',(40.,-0.3,-0.42));
#17941=CARTESIAN_POINT('',(-0.1,-0.3,-0.42));
#17942=CARTESIAN_POINT('',(40.,-0.12,-0.24));
#17943=CARTESIAN_POINT('Origin',(-0.1,0.3,-0.42));
#17944=CARTESIAN_POINT('',(0.,0.3,-0.42));
#17945=CARTESIAN_POINT('',(0.,0.15,-0.42));
#17946=CARTESIAN_POINT('',(40.,0.3,-0.42));
#17947=CARTESIAN_POINT('',(-0.1,0.3,-0.42));
#17948=CARTESIAN_POINT('',(40.,0.15,-0.42));
#17949=CARTESIAN_POINT('Origin',(-0.1,0.55,-0.67));
#17950=CARTESIAN_POINT('',(0.,0.55,-0.67));
#17951=CARTESIAN_POINT('',(0.,0.245,-0.365));
#17952=CARTESIAN_POINT('',(40.,0.55,-0.67));
#17953=CARTESIAN_POINT('',(-0.1,0.55,-0.67));
#17954=CARTESIAN_POINT('',(40.,0.245,-0.365));
#17955=CARTESIAN_POINT('Origin',(-0.1,0.55,-0.82));
#17956=CARTESIAN_POINT('',(0.,0.55,-0.82));
#17957=CARTESIAN_POINT('',(0.,0.55,-0.41));
#17958=CARTESIAN_POINT('',(40.,0.55,-0.82));
#17959=CARTESIAN_POINT('',(-0.1,0.55,-0.82));
#17960=CARTESIAN_POINT('',(40.,0.55,-0.41));
#17961=CARTESIAN_POINT('Origin',(-0.1,0.3,-0.82));
#17962=CARTESIAN_POINT('',(0.,0.3,-0.82));
#17963=CARTESIAN_POINT('',(0.,0.15,-0.82));
#17964=CARTESIAN_POINT('',(40.,0.3,-0.82));
#17965=CARTESIAN_POINT('',(-0.1,0.3,-0.82));
#17966=CARTESIAN_POINT('',(40.,0.15,-0.82));
#17967=CARTESIAN_POINT('Origin',(-0.1,0.3,-1.05));
#17968=CARTESIAN_POINT('',(0.,0.3,-1.));
#17969=CARTESIAN_POINT('',(0.,0.3,-0.525));
#17970=CARTESIAN_POINT('',(40.,0.3,-1.));
#17971=CARTESIAN_POINT('',(-0.05,0.3,-1.));
#17972=CARTESIAN_POINT('',(40.,0.3,-0.525));
#17973=CARTESIAN_POINT('Origin',(-0.1,-0.82,0.3));
#17974=CARTESIAN_POINT('',(0.,-0.82,0.3));
#17975=CARTESIAN_POINT('',(0.,-1.,0.3));
#17976=CARTESIAN_POINT('',(0.,-0.41,0.3));
#17977=CARTESIAN_POINT('',(40.,-0.82,0.3));
#17978=CARTESIAN_POINT('',(-0.1,-0.82,0.3));
#17979=CARTESIAN_POINT('',(40.,-1.,0.3));
#17980=CARTESIAN_POINT('',(40.,-0.41,0.3));
#17981=CARTESIAN_POINT('',(-0.05,-1.,0.3));
#17982=CARTESIAN_POINT('Origin',(-0.1,-0.82,0.55));
#17983=CARTESIAN_POINT('',(0.,-0.82,0.55));
#17984=CARTESIAN_POINT('',(0.,-0.82,0.275));
#17985=CARTESIAN_POINT('',(40.,-0.82,0.55));
#17986=CARTESIAN_POINT('',(-0.1,-0.82,0.55));
#17987=CARTESIAN_POINT('',(40.,-0.82,0.275));
#17988=CARTESIAN_POINT('Origin',(-0.1,-0.67,0.55));
#17989=CARTESIAN_POINT('',(0.,-0.67,0.55));
#17990=CARTESIAN_POINT('',(0.,-0.335,0.55));
#17991=CARTESIAN_POINT('',(40.,-0.67,0.55));
#17992=CARTESIAN_POINT('',(-0.1,-0.67,0.55));
#17993=CARTESIAN_POINT('',(40.,-0.335,0.55));
#17994=CARTESIAN_POINT('Origin',(-0.1,-0.42,0.3));
#17995=CARTESIAN_POINT('',(0.,-0.42,0.3));
#17996=CARTESIAN_POINT('',(-6.93889390390723E-18,-0.24,0.12));
#17997=CARTESIAN_POINT('',(40.,-0.42,0.3));
#17998=CARTESIAN_POINT('',(-0.1,-0.42,0.3));
#17999=CARTESIAN_POINT('',(40.,-0.24,0.12));
#18000=CARTESIAN_POINT('Origin',(-0.1,-0.42,-0.3));
#18001=CARTESIAN_POINT('',(0.,-0.42,-0.3));
#18002=CARTESIAN_POINT('',(0.,-0.42,-0.15));
#18003=CARTESIAN_POINT('',(40.,-0.42,-0.3));
#18004=CARTESIAN_POINT('',(-0.1,-0.42,-0.3));
#18005=CARTESIAN_POINT('',(40.,-0.42,-0.15));
#18006=CARTESIAN_POINT('Origin',(-0.1,-0.67,-0.55));
#18007=CARTESIAN_POINT('',(0.,-0.67,-0.55));
#18008=CARTESIAN_POINT('',(0.,-0.365,-0.245));
#18009=CARTESIAN_POINT('',(40.,-0.67,-0.55));
#18010=CARTESIAN_POINT('',(-0.1,-0.67,-0.55));
#18011=CARTESIAN_POINT('',(40.,-0.365,-0.245));
#18012=CARTESIAN_POINT('Origin',(-0.1,-0.82,-0.55));
#18013=CARTESIAN_POINT('',(0.,-0.82,-0.55));
#18014=CARTESIAN_POINT('',(0.,-0.41,-0.55));
#18015=CARTESIAN_POINT('',(40.,-0.82,-0.55));
#18016=CARTESIAN_POINT('',(-0.1,-0.82,-0.55));
#18017=CARTESIAN_POINT('',(40.,-0.41,-0.55));
#18018=CARTESIAN_POINT('Origin',(-0.1,-0.82,-0.3));
#18019=CARTESIAN_POINT('',(0.,-0.82,-0.3));
#18020=CARTESIAN_POINT('',(0.,-0.82,-0.15));
#18021=CARTESIAN_POINT('',(40.,-0.82,-0.3));
#18022=CARTESIAN_POINT('',(-0.1,-0.82,-0.3));
#18023=CARTESIAN_POINT('',(40.,-0.82,-0.15));
#18024=CARTESIAN_POINT('Origin',(-0.1,-1.05,-0.3));
#18025=CARTESIAN_POINT('',(0.,-1.,-0.3));
#18026=CARTESIAN_POINT('',(0.,-0.525,-0.3));
#18027=CARTESIAN_POINT('',(40.,-1.,-0.3));
#18028=CARTESIAN_POINT('',(-0.05,-1.,-0.3));
#18029=CARTESIAN_POINT('',(40.,-0.525,-0.3));
#18030=CARTESIAN_POINT('Origin',(-0.1,0.3,0.82));
#18031=CARTESIAN_POINT('',(0.,0.3,0.82));
#18032=CARTESIAN_POINT('',(0.,0.3,1.));
#18033=CARTESIAN_POINT('',(0.,0.3,0.41));
#18034=CARTESIAN_POINT('',(40.,0.3,0.82));
#18035=CARTESIAN_POINT('',(-0.1,0.3,0.82));
#18036=CARTESIAN_POINT('',(40.,0.3,1.));
#18037=CARTESIAN_POINT('',(40.,0.3,0.41));
#18038=CARTESIAN_POINT('',(-0.05,0.3,1.));
#18039=CARTESIAN_POINT('Origin',(-0.1,0.55,0.82));
#18040=CARTESIAN_POINT('',(0.,0.55,0.82));
#18041=CARTESIAN_POINT('',(0.,0.275,0.82));
#18042=CARTESIAN_POINT('',(40.,0.55,0.82));
#18043=CARTESIAN_POINT('',(-0.1,0.55,0.82));
#18044=CARTESIAN_POINT('',(40.,0.275,0.82));
#18045=CARTESIAN_POINT('Origin',(-0.1,0.55,0.67));
#18046=CARTESIAN_POINT('',(0.,0.55,0.67));
#18047=CARTESIAN_POINT('',(0.,0.55,0.335));
#18048=CARTESIAN_POINT('',(40.,0.55,0.67));
#18049=CARTESIAN_POINT('',(-0.1,0.55,0.67));
#18050=CARTESIAN_POINT('',(40.,0.55,0.335));
#18051=CARTESIAN_POINT('Origin',(-0.1,0.3,0.42));
#18052=CARTESIAN_POINT('',(0.,0.3,0.42));
#18053=CARTESIAN_POINT('',(6.93889390390723E-18,0.12,0.24));
#18054=CARTESIAN_POINT('',(40.,0.3,0.42));
#18055=CARTESIAN_POINT('',(-0.1,0.3,0.42));
#18056=CARTESIAN_POINT('',(40.,0.12,0.24));
#18057=CARTESIAN_POINT('Origin',(-0.1,-0.3,0.42));
#18058=CARTESIAN_POINT('',(0.,-0.3,0.42));
#18059=CARTESIAN_POINT('',(0.,-0.15,0.42));
#18060=CARTESIAN_POINT('',(40.,-0.3,0.42));
#18061=CARTESIAN_POINT('',(-0.1,-0.3,0.42));
#18062=CARTESIAN_POINT('',(40.,-0.15,0.42));
#18063=CARTESIAN_POINT('Origin',(-0.1,-0.55,0.67));
#18064=CARTESIAN_POINT('',(0.,-0.55,0.67));
#18065=CARTESIAN_POINT('',(6.93889390390723E-18,-0.245,0.365));
#18066=CARTESIAN_POINT('',(40.,-0.55,0.67));
#18067=CARTESIAN_POINT('',(-0.1,-0.55,0.67));
#18068=CARTESIAN_POINT('',(40.,-0.245,0.365));
#18069=CARTESIAN_POINT('Origin',(-0.1,-0.55,0.82));
#18070=CARTESIAN_POINT('',(0.,-0.55,0.82));
#18071=CARTESIAN_POINT('',(0.,-0.55,0.41));
#18072=CARTESIAN_POINT('',(40.,-0.55,0.82));
#18073=CARTESIAN_POINT('',(-0.1,-0.55,0.82));
#18074=CARTESIAN_POINT('',(40.,-0.55,0.41));
#18075=CARTESIAN_POINT('Origin',(-0.1,-0.3,0.82));
#18076=CARTESIAN_POINT('',(0.,-0.3,0.82));
#18077=CARTESIAN_POINT('',(0.,-0.15,0.82));
#18078=CARTESIAN_POINT('',(40.,-0.3,0.82));
#18079=CARTESIAN_POINT('',(-0.1,-0.3,0.82));
#18080=CARTESIAN_POINT('',(40.,-0.15,0.82));
#18081=CARTESIAN_POINT('Origin',(-0.1,-0.3,1.05));
#18082=CARTESIAN_POINT('',(0.,-0.3,1.));
#18083=CARTESIAN_POINT('',(0.,-0.3,0.525));
#18084=CARTESIAN_POINT('',(40.,-0.3,1.));
#18085=CARTESIAN_POINT('',(-0.05,-0.3,1.));
#18086=CARTESIAN_POINT('',(40.,-0.3,0.525));
#18087=CARTESIAN_POINT('Origin',(-0.1,0.,0.));
#18088=CARTESIAN_POINT('',(0.,-2.57175827820944E-17,0.21));
#18089=CARTESIAN_POINT('Origin',(0.,0.,0.));
#18090=CARTESIAN_POINT('',(40.,2.57175827820944E-17,0.21));
#18091=CARTESIAN_POINT('',(-0.1,-2.57175827820944E-17,0.21));
#18092=CARTESIAN_POINT('Origin',(40.,0.,0.));
#18093=CARTESIAN_POINT('Origin',(0.,1.,-1.));
#18094=CARTESIAN_POINT('',(0.,1.,1.));
#18095=CARTESIAN_POINT('',(0.,1.,-1.));
#18096=CARTESIAN_POINT('',(40.,1.,1.));
#18097=CARTESIAN_POINT('',(0.,1.,1.));
#18098=CARTESIAN_POINT('',(40.,1.,-1.));
#18099=CARTESIAN_POINT('Origin',(0.,1.,-1.));
#18100=CARTESIAN_POINT('',(40.,1.,-1.));
#18101=CARTESIAN_POINT('',(40.,1.,-1.));
#18102=CARTESIAN_POINT('',(0.,1.,-1.));
#18103=CARTESIAN_POINT('',(0.,1.,-1.));
#18104=CARTESIAN_POINT('',(0.,1.,-1.));
#18105=CARTESIAN_POINT('Origin',(0.,-1.,-1.));
#18106=CARTESIAN_POINT('',(0.,-1.,-1.));
#18107=CARTESIAN_POINT('',(40.,-1.,-1.));
#18108=CARTESIAN_POINT('Origin',(0.,-1.,-1.));
#18109=CARTESIAN_POINT('',(40.,-1.,-1.));
#18110=CARTESIAN_POINT('',(40.,-1.,-1.));
#18111=CARTESIAN_POINT('',(0.,-1.,-1.));
#18112=CARTESIAN_POINT('',(0.,-1.,-1.));
#18113=CARTESIAN_POINT('',(0.,-1.,-1.));
#18114=CARTESIAN_POINT('Origin',(0.,-1.,1.));
#18115=CARTESIAN_POINT('',(0.,-1.,1.));
#18116=CARTESIAN_POINT('',(40.,-1.,1.));
#18117=CARTESIAN_POINT('Origin',(0.,-1.,1.));
#18118=CARTESIAN_POINT('',(40.,-1.,1.));
#18119=CARTESIAN_POINT('',(40.,-1.,1.));
#18120=CARTESIAN_POINT('',(0.,-1.,1.));
#18121=CARTESIAN_POINT('',(0.,-1.,1.));
#18122=CARTESIAN_POINT('',(0.,-1.,1.));
#18123=CARTESIAN_POINT('Origin',(0.,1.,1.));
#18124=CARTESIAN_POINT('',(0.,1.,1.));
#18125=CARTESIAN_POINT('',(40.,1.,1.));
#18126=CARTESIAN_POINT('Origin',(0.,1.,1.));
#18127=CARTESIAN_POINT('',(40.,1.,1.));
#18128=CARTESIAN_POINT('',(0.,1.,1.));
#18129=CARTESIAN_POINT('Origin',(40.,0.,0.));
#18130=CARTESIAN_POINT('Origin',(0.,0.,0.));
#20011=UNCERTAINTY_MEASURE_WITH_UNIT(LENGTH_MEASURE(0.001),#20097,
'DISTANCE_ACCURACY_VALUE',
'Maximum model space distance between geometric entities at asserted c
onnectivities');
#20042=UNCERTAINTY_MEASURE_WITH_UNIT(LENGTH_MEASURE(0.001),#20097,
'DISTANCE_ACCURACY_VALUE',
'Maximum model space distance between geometric entities at asserted c
onnectivities');
#20065=(
GEOMETRIC_REPRESENTATION_CONTEXT(3)
GLOBAL_UNCERTAINTY_ASSIGNED_CONTEXT((#20011))
GLOBAL_UNIT_ASSIGNED_CONTEXT((#20097,#20099,#20100))
REPRESENTATION_CONTEXT('','3D')
);
#20096=(
GEOMETRIC_REPRESENTATION_CONTEXT(3)
GLOBAL_UNCERTAINTY_ASSIGNED_CONTEXT((#20042))
GLOBAL_UNIT_ASSIGNED_CONTEXT((#20097,#20099,#20100))
REPRESENTATION_CONTEXT('','3D')
);
#20097=(
LENGTH_UNIT()
NAMED_UNIT(*)
SI_UNIT(.CENTI.,.METRE.)
);
#20099=(
NAMED_UNIT(*)
PLANE_ANGLE_UNIT()
SI_UNIT($,.RADIAN.)
);
#20100=(
NAMED_UNIT(*)
SI_UNIT($,.STERADIAN.)
SOLID_ANGLE_UNIT()
);
#20123=SHAPE_DEFINITION_REPRESENTATION(#20181,#20334);
#20181=PRODUCT_DEFINITION_SHAPE('',$,#20388);
#20334=SHAPE_REPRESENTATION('',(#12050),#20065);
#20365=PRODUCT_DEFINITION_CONTEXT('part definition',#20526,'design');
#20388=PRODUCT_DEFINITION('Slotted Extrusion - 20 x 20 x 400 mm',
'Slotted Extrusion - 20 x 20 x 400 mm',#20441,#20365);
#20441=PRODUCT_DEFINITION_FORMATION('',$,#20550);
#20526=APPLICATION_CONTEXT(
'Core Data for Automotive Mechanical Design Process');
#20527=PRODUCT_CONTEXT('part definition',#20526,'mechanical');
#20550=PRODUCT('Slotted Extrusion - 20 x 20 x 400 mm',
'Slotted Extrusion - 20 x 20 x 400 mm',
'Slotted Extrusion - 20 x 20 x 400 mm',(#20527));
#20630=COLOUR_RGB('Light Blue',0.38,0.62,0.78);
#20631=FILL_AREA_STYLE_COLOUR('',#20630);
#20632=FILL_AREA_STYLE('',(#20631));
#20633=SURFACE_STYLE_FILL_AREA(#20632);
#20634=SURFACE_SIDE_STYLE('',(#20633));
#20635=SURFACE_STYLE_USAGE(.BOTH.,#20634);
#20636=PRESENTATION_STYLE_ASSIGNMENT((#20635));
ENDSEC;
END-ISO-10303-21;
